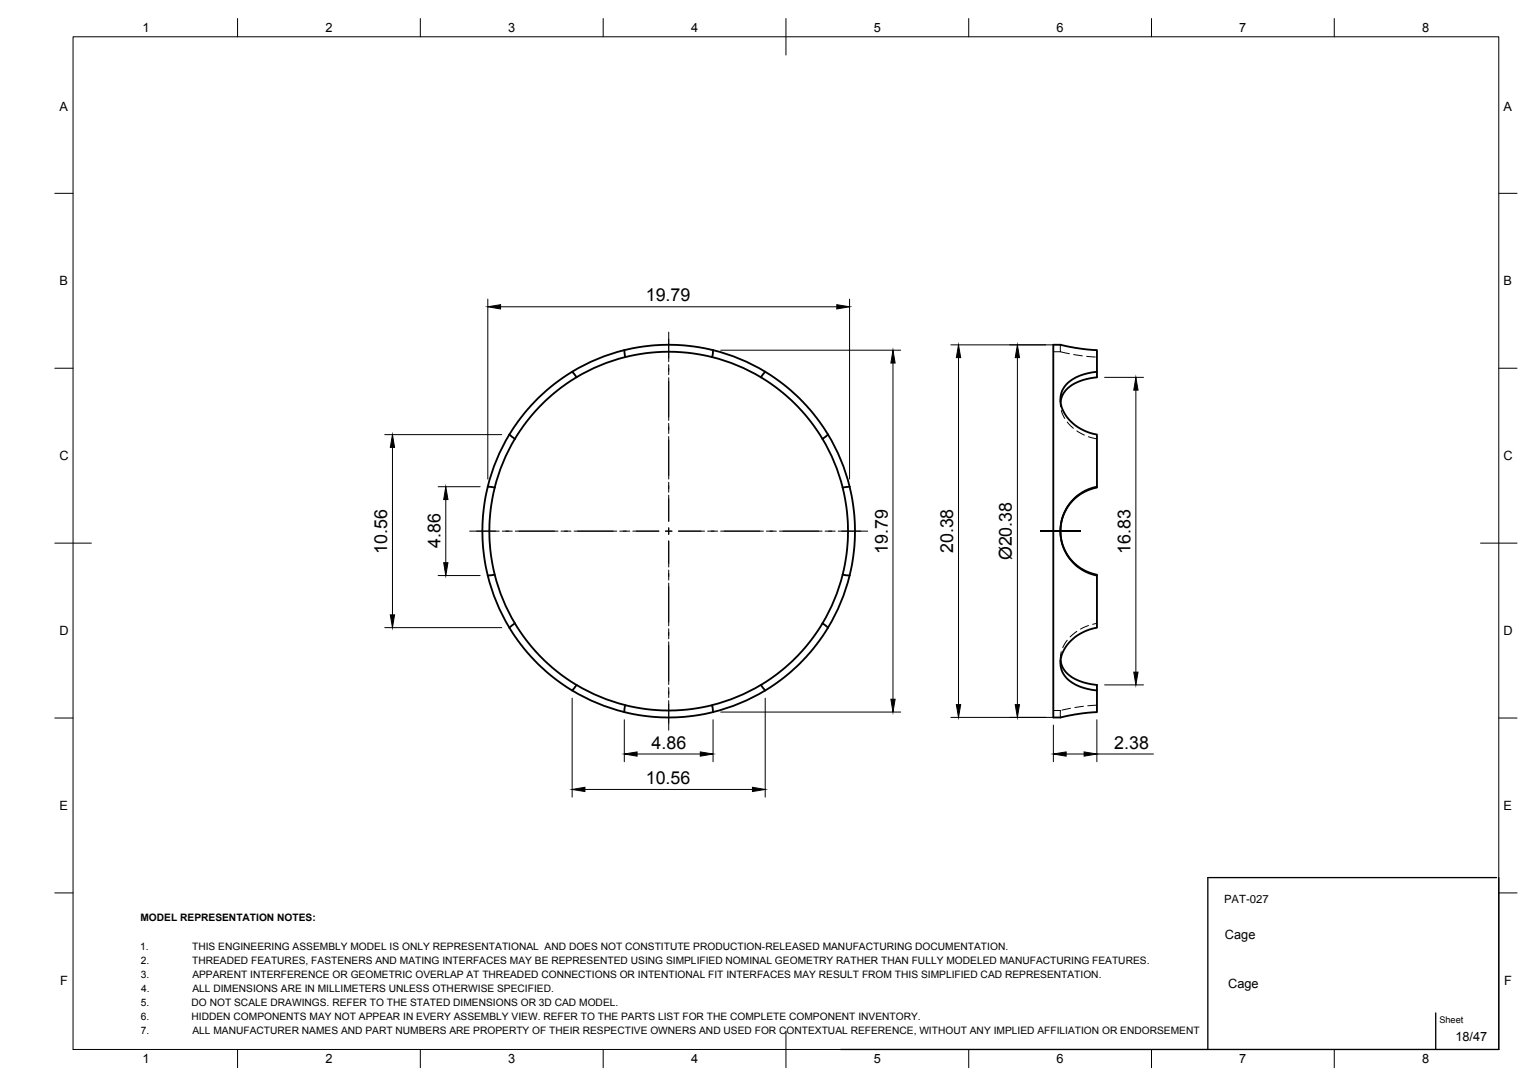
ISO-10303-21;
HEADER;
/* Generated by software containing ST-Developer
 * from STEP Tools, Inc. (www.steptools.com) 
 */

FILE_DESCRIPTION(
/* description */ ('Crank-driven oscillating fan base (mechanism only)'),

/* implementation_level */ '2;1');

FILE_NAME(
/* name */ 'Cage.step',
/* time_stamp */ '2026-10-28T03:25:00-07:00',
/* author */ (''),
/* organization */ (''),
/* preprocessor_version */ 'ST-DEVELOPER v20.2',
/* originating_system */ 'Autodesk Translation Framework v15.17.0.0',
/* authorisation */ '');

FILE_SCHEMA (('AUTOMOTIVE_DESIGN { 1 0 10303 214 3 1 1 }'));
ENDSEC;

DATA;
#10=MECHANICAL_DESIGN_GEOMETRIC_PRESENTATION_REPRESENTATION('',(#456),#11916);
#283=SPHERICAL_SURFACE('',#6888,0.247676);
#284=SPHERICAL_SURFACE('',#6904,0.247676);
#285=SPHERICAL_SURFACE('',#6909,0.247676);
#286=SPHERICAL_SURFACE('',#6914,0.247676);
#287=SPHERICAL_SURFACE('',#6919,0.247676);
#288=SPHERICAL_SURFACE('',#6924,0.247676);
#289=SPHERICAL_SURFACE('',#6929,0.247676);
#290=SPHERICAL_SURFACE('',#6937,0.247676);
#324=B_SPLINE_CURVE_WITH_KNOTS('',3,(#10274,#10275,#10276,#10277,#10278,
#10279,#10280,#10281,#10282,#10283,#10284,#10285,#10286,#10287,#10288,#10289,
#10290,#10291,#10292,#10293,#10294,#10295),.UNSPECIFIED.,.F.,.F.,(4,2,2,
2,2,2,2,2,2,2,4),(0.0473477652366656,0.126350602536658,0.189525903804987,
0.252701205073317,0.313298422430275,0.373895639787233,0.434492857144191,
0.495090074501149,0.558265375769478,0.621440677037807,0.7004435143378),
 .UNSPECIFIED.);
#325=B_SPLINE_CURVE_WITH_KNOTS('',3,(#10299,#10300,#10301,#10302,#10303,
#10304,#10305,#10306,#10307,#10308,#10309,#10310,#10311,#10312,#10313,#10314,
#10315,#10316,#10317,#10318,#10319,#10320),.UNSPECIFIED.,.F.,.F.,(4,2,2,
2,2,2,2,2,2,2,4),(0.0464897534940957,0.0852567806515119,0.170513561303024,
0.246687263103517,0.308657850341199,0.370628437578881,0.432599024816563,
0.494569612054245,0.570743313854739,0.656000094506251,0.694767121663666),
 .UNSPECIFIED.);
#326=B_SPLINE_CURVE_WITH_KNOTS('',3,(#10326,#10327,#10328,#10329,#10330,
#10331,#10332,#10333,#10334,#10335,#10336,#10337,#10338,#10339,#10340,#10341,
#10342,#10343,#10344,#10345,#10346,#10347),.UNSPECIFIED.,.F.,.F.,(4,2,2,
2,2,2,2,2,2,2,4),(0.0464897534940957,0.0852567806515118,0.170513561303024,
0.246687263103517,0.308657850341199,0.370628437578881,0.432599024816563,
0.494569612054245,0.570743313854738,0.65600009450625,0.694767121663666),
 .UNSPECIFIED.);
#327=B_SPLINE_CURVE_WITH_KNOTS('',3,(#10351,#10352,#10353,#10354,#10355,
#10356,#10357,#10358,#10359,#10360,#10361,#10362,#10363,#10364,#10365,#10366,
#10367,#10368,#10369,#10370,#10371,#10372),.UNSPECIFIED.,.F.,.F.,(4,2,2,
2,2,2,2,2,2,2,4),(0.0464897534940957,0.0852567806515119,0.170513561303024,
0.246687263103517,0.308657850341199,0.370628437578881,0.432599024816563,
0.494569612054245,0.570743313854739,0.656000094506251,0.694767121663666),
 .UNSPECIFIED.);
#328=B_SPLINE_CURVE_WITH_KNOTS('',3,(#10376,#10377,#10378,#10379,#10380,
#10381,#10382,#10383,#10384,#10385,#10386,#10387),.UNSPECIFIED.,.F.,.F.,
(4,2,2,2,2,4),(0.0464897534940957,0.0852567806515119,0.170513561303024,
0.246687263103517,0.308657850341199,0.370628437578881),.UNSPECIFIED.);
#329=B_SPLINE_CURVE_WITH_KNOTS('',3,(#10392,#10393,#10394,#10395,#10396,
#10397,#10398,#10399,#10400,#10401,#10402,#10403),.UNSPECIFIED.,.F.,.F.,
(4,2,2,2,2,4),(0.370628437578881,0.432599024816563,0.494569612054245,0.570743313854738,
0.65600009450625,0.694767121663666),.UNSPECIFIED.);
#330=B_SPLINE_CURVE_WITH_KNOTS('',3,(#10407,#10408,#10409,#10410,#10411,
#10412,#10413,#10414,#10415,#10416,#10417,#10418,#10419,#10420,#10421,#10422,
#10423,#10424,#10425,#10426,#10427,#10428),.UNSPECIFIED.,.F.,.F.,(4,2,2,
2,2,2,2,2,2,2,4),(0.0464897534940957,0.0852567806515121,0.170513561303024,
0.246687263103518,0.308657850341199,0.370628437578881,0.432599024816563,
0.494569612054245,0.570743313854738,0.65600009450625,0.694767121663666),
 .UNSPECIFIED.);
#331=B_SPLINE_CURVE_WITH_KNOTS('',3,(#10432,#10433,#10434,#10435,#10436,
#10437,#10438,#10439,#10440,#10441,#10442,#10443,#10444,#10445,#10446,#10447,
#10448,#10449,#10450,#10451,#10452,#10453),.UNSPECIFIED.,.F.,.F.,(4,2,2,
2,2,2,2,2,2,2,4),(0.0464897534940957,0.0852567806515119,0.170513561303024,
0.246687263103517,0.308657850341199,0.370628437578881,0.432599024816563,
0.494569612054245,0.570743313854738,0.65600009450625,0.694767121663667),
 .UNSPECIFIED.);
#332=B_SPLINE_CURVE_WITH_KNOTS('',3,(#10457,#10458,#10459,#10460,#10461,
#10462,#10463,#10464,#10465,#10466,#10467,#10468,#10469,#10470,#10471,#10472,
#10473,#10474,#10475,#10476,#10477,#10478),.UNSPECIFIED.,.F.,.F.,(4,2,2,
2,2,2,2,2,2,2,4),(0.0464897534940957,0.0852567806515119,0.170513561303024,
0.246687263103517,0.308657850341199,0.370628437578881,0.432599024816563,
0.494569612054245,0.570743313854738,0.65600009450625,0.694767121663666),
 .UNSPECIFIED.);
#333=B_SPLINE_CURVE_WITH_KNOTS('',3,(#10482,#10483,#10484,#10485,#10486,
#10487,#10488,#10489,#10490,#10491,#10492,#10493,#10494,#10495,#10496,#10497,
#10498,#10499,#10500,#10501,#10502,#10503),.UNSPECIFIED.,.F.,.F.,(4,2,2,
2,2,2,2,2,2,2,4),(0.0464897534940957,0.0852567806515119,0.170513561303024,
0.246687263103517,0.308657850341199,0.370628437578881,0.432599024816563,
0.494569612054245,0.570743313854739,0.656000094506251,0.694767121663667),
 .UNSPECIFIED.);
#334=B_SPLINE_CURVE_WITH_KNOTS('',3,(#10511,#10512,#10513,#10514,#10515,
#10516,#10517,#10518,#10519,#10520,#10521,#10522,#10523,#10524,#10525,#10526,
#10527,#10528,#10529,#10530,#10531,#10532),.UNSPECIFIED.,.F.,.F.,(4,2,2,
2,2,2,2,2,2,2,4),(0.0473477652366656,0.126350602536658,0.189525903804987,
0.252701205073316,0.313298422430274,0.373895639787232,0.434492857144191,
0.495090074501149,0.558265375769478,0.621440677037807,0.7004435143378),
 .UNSPECIFIED.);
#335=B_SPLINE_CURVE_WITH_KNOTS('',3,(#10540,#10541,#10542,#10543,#10544,
#10545,#10546,#10547,#10548,#10549,#10550,#10551,#10552,#10553,#10554,#10555,
#10556,#10557,#10558,#10559,#10560,#10561),.UNSPECIFIED.,.F.,.F.,(4,2,2,
2,2,2,2,2,2,2,4),(0.0473477652366656,0.126350602536658,0.189525903804987,
0.252701205073317,0.313298422430275,0.373895639787233,0.434492857144191,
0.495090074501149,0.558265375769478,0.621440677037807,0.7004435143378),
 .UNSPECIFIED.);
#336=B_SPLINE_CURVE_WITH_KNOTS('',3,(#10570,#10571,#10572,#10573,#10574,
#10575,#10576,#10577,#10578,#10579,#10580,#10581),.UNSPECIFIED.,.F.,.F.,
(4,2,2,2,2,4),(0.0473477652366656,0.126350602536658,0.189525903804987,0.252701205073316,
0.313298422430275,0.373895639787233),.UNSPECIFIED.);
#337=B_SPLINE_CURVE_WITH_KNOTS('',3,(#10583,#10584,#10585,#10586,#10587,
#10588,#10589,#10590,#10591,#10592,#10593,#10594),.UNSPECIFIED.,.F.,.F.,
(4,2,2,2,2,4),(0.373895639787233,0.434492857144191,0.495090074501149,0.558265375769478,
0.621440677037807,0.7004435143378),.UNSPECIFIED.);
#338=B_SPLINE_CURVE_WITH_KNOTS('',3,(#10601,#10602,#10603,#10604,#10605,
#10606,#10607,#10608,#10609,#10610,#10611,#10612,#10613,#10614,#10615,#10616,
#10617,#10618,#10619,#10620,#10621,#10622),.UNSPECIFIED.,.F.,.F.,(4,2,2,
2,2,2,2,2,2,2,4),(0.0473477652366656,0.126350602536658,0.189525903804987,
0.252701205073316,0.313298422430275,0.373895639787233,0.434492857144191,
0.495090074501149,0.558265375769478,0.621440677037807,0.7004435143378),
 .UNSPECIFIED.);
#339=B_SPLINE_CURVE_WITH_KNOTS('',3,(#10630,#10631,#10632,#10633,#10634,
#10635,#10636,#10637,#10638,#10639,#10640,#10641,#10642,#10643,#10644,#10645,
#10646,#10647,#10648,#10649,#10650,#10651),.UNSPECIFIED.,.F.,.F.,(4,2,2,
2,2,2,2,2,2,2,4),(0.0473477652366656,0.126350602536658,0.189525903804987,
0.252701205073317,0.313298422430275,0.373895639787233,0.434492857144191,
0.495090074501149,0.558265375769478,0.621440677037807,0.7004435143378),
 .UNSPECIFIED.);
#340=B_SPLINE_CURVE_WITH_KNOTS('',3,(#10659,#10660,#10661,#10662,#10663,
#10664,#10665,#10666,#10667,#10668,#10669,#10670,#10671,#10672,#10673,#10674,
#10675,#10676,#10677,#10678,#10679,#10680),.UNSPECIFIED.,.F.,.F.,(4,2,2,
2,2,2,2,2,2,2,4),(0.0473477652366656,0.126350602536658,0.189525903804987,
0.252701205073316,0.313298422430275,0.373895639787233,0.434492857144191,
0.495090074501149,0.558265375769478,0.621440677037807,0.7004435143378),
 .UNSPECIFIED.);
#341=B_SPLINE_CURVE_WITH_KNOTS('',3,(#10689,#10690,#10691,#10692,#10693,
#10694,#10695,#10696,#10697,#10698,#10699,#10700,#10701,#10702,#10703,#10704,
#10705,#10706,#10707,#10708,#10709,#10710),.UNSPECIFIED.,.F.,.F.,(4,2,2,
2,2,2,2,2,2,2,4),(0.0473477652366656,0.126350602536658,0.189525903804987,
0.252701205073317,0.313298422430275,0.373895639787233,0.434492857144191,
0.495090074501149,0.558265375769478,0.621440677037807,0.7004435143378),
 .UNSPECIFIED.);
#369=SHAPE_REPRESENTATION_RELATIONSHIP('SRR','None',#12094,#409);
#409=ADVANCED_BREP_SHAPE_REPRESENTATION('',(#503),#11885);
#456=STYLED_ITEM('',(#12375),#503);
#503=MANIFOLD_SOLID_BREP('Continuous crown cage',#6087);
#611=FACE_BOUND('',#1508,.T.);
#757=PLANE('',#6901);
#758=PLANE('',#6906);
#759=PLANE('',#6911);
#760=PLANE('',#6916);
#761=PLANE('',#6921);
#762=PLANE('',#6926);
#763=PLANE('',#6935);
#764=PLANE('',#6939);
#765=PLANE('',#6940);
#1034=FACE_OUTER_BOUND('',#1490,.T.);
#1035=FACE_OUTER_BOUND('',#1491,.T.);
#1036=FACE_OUTER_BOUND('',#1492,.T.);
#1037=FACE_OUTER_BOUND('',#1493,.T.);
#1038=FACE_OUTER_BOUND('',#1494,.T.);
#1039=FACE_OUTER_BOUND('',#1495,.T.);
#1040=FACE_OUTER_BOUND('',#1496,.T.);
#1041=FACE_OUTER_BOUND('',#1497,.T.);
#1042=FACE_OUTER_BOUND('',#1498,.T.);
#1043=FACE_OUTER_BOUND('',#1499,.T.);
#1044=FACE_OUTER_BOUND('',#1500,.T.);
#1045=FACE_OUTER_BOUND('',#1501,.T.);
#1046=FACE_OUTER_BOUND('',#1502,.T.);
#1047=FACE_OUTER_BOUND('',#1503,.T.);
#1048=FACE_OUTER_BOUND('',#1504,.T.);
#1049=FACE_OUTER_BOUND('',#1505,.T.);
#1050=FACE_OUTER_BOUND('',#1506,.T.);
#1051=FACE_OUTER_BOUND('',#1507,.T.);
#1052=FACE_OUTER_BOUND('',#1509,.T.);
#1490=EDGE_LOOP('',(#4684,#4685,#4686,#4687));
#1491=EDGE_LOOP('',(#4688,#4689,#4690,#4691,#4692,#4693,#4694,#4695,#4696,
#4697,#4698,#4699,#4700,#4701,#4702,#4703,#4704,#4705,#4706,#4707));
#1492=EDGE_LOOP('',(#4708,#4709,#4710,#4711));
#1493=EDGE_LOOP('',(#4712,#4713,#4714,#4715));
#1494=EDGE_LOOP('',(#4716,#4717,#4718,#4719));
#1495=EDGE_LOOP('',(#4720,#4721,#4722,#4723));
#1496=EDGE_LOOP('',(#4724,#4725,#4726,#4727));
#1497=EDGE_LOOP('',(#4728,#4729,#4730,#4731,#4732,#4733));
#1498=EDGE_LOOP('',(#4734,#4735,#4736,#4737));
#1499=EDGE_LOOP('',(#4738,#4739,#4740,#4741));
#1500=EDGE_LOOP('',(#4742,#4743,#4744,#4745));
#1501=EDGE_LOOP('',(#4746,#4747,#4748,#4749));
#1502=EDGE_LOOP('',(#4750,#4751,#4752,#4753));
#1503=EDGE_LOOP('',(#4754,#4755,#4756,#4757));
#1504=EDGE_LOOP('',(#4758,#4759,#4760,#4761,#4762,#4763,#4764,#4765,#4766,
#4767,#4768,#4769,#4770,#4771,#4772,#4773,#4774,#4775,#4776,#4777));
#1505=EDGE_LOOP('',(#4778,#4779,#4780,#4781));
#1506=EDGE_LOOP('',(#4782,#4783,#4784,#4785));
#1507=EDGE_LOOP('',(#4786));
#1508=EDGE_LOOP('',(#4787));
#1509=EDGE_LOOP('',(#4788,#4789,#4790,#4791));
#1933=LINE('',#10389,#2266);
#1934=LINE('',#10685,#2267);
#2266=VECTOR('',#8218,1.019052);
#2267=VECTOR('',#8295,0.980948);
#2629=CIRCLE('',#6889,0.243053047864041);
#2630=CIRCLE('',#6890,0.243053047864041);
#2631=CIRCLE('',#6892,1.019052);
#2632=CIRCLE('',#6893,1.019052);
#2633=CIRCLE('',#6894,1.019052);
#2634=CIRCLE('',#6895,1.019052);
#2635=CIRCLE('',#6896,1.019052);
#2636=CIRCLE('',#6897,1.019052);
#2637=CIRCLE('',#6898,1.019052);
#2638=CIRCLE('',#6899,1.019052);
#2639=CIRCLE('',#6900,1.019052);
#2640=CIRCLE('',#6902,0.980948);
#2641=CIRCLE('',#6903,0.243053047864041);
#2642=CIRCLE('',#6905,0.243053047864041);
#2643=CIRCLE('',#6907,0.980948);
#2644=CIRCLE('',#6908,0.243053047864041);
#2645=CIRCLE('',#6910,0.243053047864041);
#2646=CIRCLE('',#6912,0.980948);
#2647=CIRCLE('',#6913,0.243053047864041);
#2648=CIRCLE('',#6915,0.243053047864041);
#2649=CIRCLE('',#6917,0.980948);
#2650=CIRCLE('',#6918,0.243053047864041);
#2651=CIRCLE('',#6920,0.243053047864041);
#2652=CIRCLE('',#6922,0.980948);
#2653=CIRCLE('',#6923,0.243053047864041);
#2654=CIRCLE('',#6925,0.243053047864041);
#2655=CIRCLE('',#6927,0.980948);
#2656=CIRCLE('',#6928,0.243053047864041);
#2657=CIRCLE('',#6930,0.243053047864041);
#2658=CIRCLE('',#6932,0.980948);
#2659=CIRCLE('',#6933,0.980948);
#2660=CIRCLE('',#6934,0.980948);
#2661=CIRCLE('',#6936,0.243053047864041);
#2662=CIRCLE('',#6938,0.243053047864041);
#3044=VERTEX_POINT('',#10272);
#3045=VERTEX_POINT('',#10273);
#3046=VERTEX_POINT('',#10296);
#3047=VERTEX_POINT('',#10298);
#3048=VERTEX_POINT('',#10323);
#3049=VERTEX_POINT('',#10325);
#3050=VERTEX_POINT('',#10348);
#3051=VERTEX_POINT('',#10350);
#3052=VERTEX_POINT('',#10373);
#3053=VERTEX_POINT('',#10375);
#3054=VERTEX_POINT('',#10388);
#3055=VERTEX_POINT('',#10391);
#3056=VERTEX_POINT('',#10404);
#3057=VERTEX_POINT('',#10406);
#3058=VERTEX_POINT('',#10429);
#3059=VERTEX_POINT('',#10431);
#3060=VERTEX_POINT('',#10454);
#3061=VERTEX_POINT('',#10456);
#3062=VERTEX_POINT('',#10479);
#3063=VERTEX_POINT('',#10481);
#3064=VERTEX_POINT('',#10506);
#3065=VERTEX_POINT('',#10510);
#3066=VERTEX_POINT('',#10535);
#3067=VERTEX_POINT('',#10539);
#3068=VERTEX_POINT('',#10564);
#3069=VERTEX_POINT('',#10568);
#3070=VERTEX_POINT('',#10569);
#3071=VERTEX_POINT('',#10596);
#3072=VERTEX_POINT('',#10600);
#3073=VERTEX_POINT('',#10625);
#3074=VERTEX_POINT('',#10629);
#3075=VERTEX_POINT('',#10654);
#3076=VERTEX_POINT('',#10658);
#3077=VERTEX_POINT('',#10683);
#3078=VERTEX_POINT('',#10686);
#3079=VERTEX_POINT('',#10688);
#3637=EDGE_CURVE('',#3044,#3045,#324,.T.);
#3638=EDGE_CURVE('',#3046,#3044,#2629,.T.);
#3639=EDGE_CURVE('',#3047,#3046,#325,.T.);
#3640=EDGE_CURVE('',#3045,#3047,#2630,.T.);
#3641=EDGE_CURVE('',#3048,#3046,#2631,.T.);
#3642=EDGE_CURVE('',#3048,#3049,#326,.T.);
#3643=EDGE_CURVE('',#3050,#3049,#2632,.T.);
#3644=EDGE_CURVE('',#3050,#3051,#327,.T.);
#3645=EDGE_CURVE('',#3052,#3051,#2633,.T.);
#3646=EDGE_CURVE('',#3052,#3053,#328,.T.);
#3647=EDGE_CURVE('',#3053,#3054,#1933,.T.);
#3648=EDGE_CURVE('',#3054,#3054,#2634,.T.);
#3649=EDGE_CURVE('',#3053,#3055,#329,.T.);
#3650=EDGE_CURVE('',#3056,#3055,#2635,.T.);
#3651=EDGE_CURVE('',#3056,#3057,#330,.T.);
#3652=EDGE_CURVE('',#3058,#3057,#2636,.T.);
#3653=EDGE_CURVE('',#3058,#3059,#331,.T.);
#3654=EDGE_CURVE('',#3060,#3059,#2637,.T.);
#3655=EDGE_CURVE('',#3060,#3061,#332,.T.);
#3656=EDGE_CURVE('',#3062,#3061,#2638,.T.);
#3657=EDGE_CURVE('',#3062,#3063,#333,.T.);
#3658=EDGE_CURVE('',#3047,#3063,#2639,.T.);
#3659=EDGE_CURVE('',#3044,#3064,#2640,.T.);
#3660=EDGE_CURVE('',#3064,#3048,#2641,.T.);
#3661=EDGE_CURVE('',#3065,#3064,#334,.T.);
#3662=EDGE_CURVE('',#3049,#3065,#2642,.T.);
#3663=EDGE_CURVE('',#3065,#3066,#2643,.T.);
#3664=EDGE_CURVE('',#3066,#3050,#2644,.T.);
#3665=EDGE_CURVE('',#3067,#3066,#335,.T.);
#3666=EDGE_CURVE('',#3051,#3067,#2645,.T.);
#3667=EDGE_CURVE('',#3067,#3068,#2646,.T.);
#3668=EDGE_CURVE('',#3068,#3052,#2647,.T.);
#3669=EDGE_CURVE('',#3069,#3070,#336,.T.);
#3670=EDGE_CURVE('',#3055,#3069,#2648,.T.);
#3671=EDGE_CURVE('',#3070,#3068,#337,.T.);
#3672=EDGE_CURVE('',#3069,#3071,#2649,.T.);
#3673=EDGE_CURVE('',#3071,#3056,#2650,.T.);
#3674=EDGE_CURVE('',#3072,#3071,#338,.T.);
#3675=EDGE_CURVE('',#3057,#3072,#2651,.T.);
#3676=EDGE_CURVE('',#3072,#3073,#2652,.T.);
#3677=EDGE_CURVE('',#3073,#3058,#2653,.T.);
#3678=EDGE_CURVE('',#3074,#3073,#339,.T.);
#3679=EDGE_CURVE('',#3059,#3074,#2654,.T.);
#3680=EDGE_CURVE('',#3074,#3075,#2655,.T.);
#3681=EDGE_CURVE('',#3075,#3060,#2656,.T.);
#3682=EDGE_CURVE('',#3076,#3075,#340,.T.);
#3683=EDGE_CURVE('',#3061,#3076,#2657,.T.);
#3684=EDGE_CURVE('',#3077,#3077,#2658,.T.);
#3685=EDGE_CURVE('',#3077,#3070,#1934,.T.);
#3686=EDGE_CURVE('',#3078,#3045,#2659,.T.);
#3687=EDGE_CURVE('',#3078,#3079,#341,.T.);
#3688=EDGE_CURVE('',#3076,#3079,#2660,.T.);
#3689=EDGE_CURVE('',#3063,#3078,#2661,.T.);
#3690=EDGE_CURVE('',#3079,#3062,#2662,.T.);
#4684=ORIENTED_EDGE('',*,*,#3637,.F.);
#4685=ORIENTED_EDGE('',*,*,#3638,.F.);
#4686=ORIENTED_EDGE('',*,*,#3639,.F.);
#4687=ORIENTED_EDGE('',*,*,#3640,.F.);
#4688=ORIENTED_EDGE('',*,*,#3639,.T.);
#4689=ORIENTED_EDGE('',*,*,#3641,.F.);
#4690=ORIENTED_EDGE('',*,*,#3642,.T.);
#4691=ORIENTED_EDGE('',*,*,#3643,.F.);
#4692=ORIENTED_EDGE('',*,*,#3644,.T.);
#4693=ORIENTED_EDGE('',*,*,#3645,.F.);
#4694=ORIENTED_EDGE('',*,*,#3646,.T.);
#4695=ORIENTED_EDGE('',*,*,#3647,.T.);
#4696=ORIENTED_EDGE('',*,*,#3648,.F.);
#4697=ORIENTED_EDGE('',*,*,#3647,.F.);
#4698=ORIENTED_EDGE('',*,*,#3649,.T.);
#4699=ORIENTED_EDGE('',*,*,#3650,.F.);
#4700=ORIENTED_EDGE('',*,*,#3651,.T.);
#4701=ORIENTED_EDGE('',*,*,#3652,.F.);
#4702=ORIENTED_EDGE('',*,*,#3653,.T.);
#4703=ORIENTED_EDGE('',*,*,#3654,.F.);
#4704=ORIENTED_EDGE('',*,*,#3655,.T.);
#4705=ORIENTED_EDGE('',*,*,#3656,.F.);
#4706=ORIENTED_EDGE('',*,*,#3657,.T.);
#4707=ORIENTED_EDGE('',*,*,#3658,.F.);
#4708=ORIENTED_EDGE('',*,*,#3638,.T.);
#4709=ORIENTED_EDGE('',*,*,#3659,.T.);
#4710=ORIENTED_EDGE('',*,*,#3660,.T.);
#4711=ORIENTED_EDGE('',*,*,#3641,.T.);
#4712=ORIENTED_EDGE('',*,*,#3661,.F.);
#4713=ORIENTED_EDGE('',*,*,#3662,.F.);
#4714=ORIENTED_EDGE('',*,*,#3642,.F.);
#4715=ORIENTED_EDGE('',*,*,#3660,.F.);
#4716=ORIENTED_EDGE('',*,*,#3662,.T.);
#4717=ORIENTED_EDGE('',*,*,#3663,.T.);
#4718=ORIENTED_EDGE('',*,*,#3664,.T.);
#4719=ORIENTED_EDGE('',*,*,#3643,.T.);
#4720=ORIENTED_EDGE('',*,*,#3665,.F.);
#4721=ORIENTED_EDGE('',*,*,#3666,.F.);
#4722=ORIENTED_EDGE('',*,*,#3644,.F.);
#4723=ORIENTED_EDGE('',*,*,#3664,.F.);
#4724=ORIENTED_EDGE('',*,*,#3666,.T.);
#4725=ORIENTED_EDGE('',*,*,#3667,.T.);
#4726=ORIENTED_EDGE('',*,*,#3668,.T.);
#4727=ORIENTED_EDGE('',*,*,#3645,.T.);
#4728=ORIENTED_EDGE('',*,*,#3669,.F.);
#4729=ORIENTED_EDGE('',*,*,#3670,.F.);
#4730=ORIENTED_EDGE('',*,*,#3649,.F.);
#4731=ORIENTED_EDGE('',*,*,#3646,.F.);
#4732=ORIENTED_EDGE('',*,*,#3668,.F.);
#4733=ORIENTED_EDGE('',*,*,#3671,.F.);
#4734=ORIENTED_EDGE('',*,*,#3670,.T.);
#4735=ORIENTED_EDGE('',*,*,#3672,.T.);
#4736=ORIENTED_EDGE('',*,*,#3673,.T.);
#4737=ORIENTED_EDGE('',*,*,#3650,.T.);
#4738=ORIENTED_EDGE('',*,*,#3674,.F.);
#4739=ORIENTED_EDGE('',*,*,#3675,.F.);
#4740=ORIENTED_EDGE('',*,*,#3651,.F.);
#4741=ORIENTED_EDGE('',*,*,#3673,.F.);
#4742=ORIENTED_EDGE('',*,*,#3675,.T.);
#4743=ORIENTED_EDGE('',*,*,#3676,.T.);
#4744=ORIENTED_EDGE('',*,*,#3677,.T.);
#4745=ORIENTED_EDGE('',*,*,#3652,.T.);
#4746=ORIENTED_EDGE('',*,*,#3678,.F.);
#4747=ORIENTED_EDGE('',*,*,#3679,.F.);
#4748=ORIENTED_EDGE('',*,*,#3653,.F.);
#4749=ORIENTED_EDGE('',*,*,#3677,.F.);
#4750=ORIENTED_EDGE('',*,*,#3679,.T.);
#4751=ORIENTED_EDGE('',*,*,#3680,.T.);
#4752=ORIENTED_EDGE('',*,*,#3681,.T.);
#4753=ORIENTED_EDGE('',*,*,#3654,.T.);
#4754=ORIENTED_EDGE('',*,*,#3655,.F.);
#4755=ORIENTED_EDGE('',*,*,#3681,.F.);
#4756=ORIENTED_EDGE('',*,*,#3682,.F.);
#4757=ORIENTED_EDGE('',*,*,#3683,.F.);
#4758=ORIENTED_EDGE('',*,*,#3684,.F.);
#4759=ORIENTED_EDGE('',*,*,#3685,.T.);
#4760=ORIENTED_EDGE('',*,*,#3671,.T.);
#4761=ORIENTED_EDGE('',*,*,#3667,.F.);
#4762=ORIENTED_EDGE('',*,*,#3665,.T.);
#4763=ORIENTED_EDGE('',*,*,#3663,.F.);
#4764=ORIENTED_EDGE('',*,*,#3661,.T.);
#4765=ORIENTED_EDGE('',*,*,#3659,.F.);
#4766=ORIENTED_EDGE('',*,*,#3637,.T.);
#4767=ORIENTED_EDGE('',*,*,#3686,.F.);
#4768=ORIENTED_EDGE('',*,*,#3687,.T.);
#4769=ORIENTED_EDGE('',*,*,#3688,.F.);
#4770=ORIENTED_EDGE('',*,*,#3682,.T.);
#4771=ORIENTED_EDGE('',*,*,#3680,.F.);
#4772=ORIENTED_EDGE('',*,*,#3678,.T.);
#4773=ORIENTED_EDGE('',*,*,#3676,.F.);
#4774=ORIENTED_EDGE('',*,*,#3674,.T.);
#4775=ORIENTED_EDGE('',*,*,#3672,.F.);
#4776=ORIENTED_EDGE('',*,*,#3669,.T.);
#4777=ORIENTED_EDGE('',*,*,#3685,.F.);
#4778=ORIENTED_EDGE('',*,*,#3640,.T.);
#4779=ORIENTED_EDGE('',*,*,#3658,.T.);
#4780=ORIENTED_EDGE('',*,*,#3689,.T.);
#4781=ORIENTED_EDGE('',*,*,#3686,.T.);
#4782=ORIENTED_EDGE('',*,*,#3657,.F.);
#4783=ORIENTED_EDGE('',*,*,#3690,.F.);
#4784=ORIENTED_EDGE('',*,*,#3687,.F.);
#4785=ORIENTED_EDGE('',*,*,#3689,.F.);
#4786=ORIENTED_EDGE('',*,*,#3648,.T.);
#4787=ORIENTED_EDGE('',*,*,#3684,.T.);
#4788=ORIENTED_EDGE('',*,*,#3683,.T.);
#4789=ORIENTED_EDGE('',*,*,#3688,.T.);
#4790=ORIENTED_EDGE('',*,*,#3690,.T.);
#4791=ORIENTED_EDGE('',*,*,#3656,.T.);
#5612=CYLINDRICAL_SURFACE('',#6891,1.019052);
#5613=CYLINDRICAL_SURFACE('',#6931,0.980948);
#5840=ADVANCED_FACE('',(#1034),#283,.F.);
#5841=ADVANCED_FACE('',(#1035),#5612,.T.);
#5842=ADVANCED_FACE('',(#1036),#757,.T.);
#5843=ADVANCED_FACE('',(#1037),#284,.F.);
#5844=ADVANCED_FACE('',(#1038),#758,.T.);
#5845=ADVANCED_FACE('',(#1039),#285,.F.);
#5846=ADVANCED_FACE('',(#1040),#759,.T.);
#5847=ADVANCED_FACE('',(#1041),#286,.F.);
#5848=ADVANCED_FACE('',(#1042),#760,.T.);
#5849=ADVANCED_FACE('',(#1043),#287,.F.);
#5850=ADVANCED_FACE('',(#1044),#761,.T.);
#5851=ADVANCED_FACE('',(#1045),#288,.F.);
#5852=ADVANCED_FACE('',(#1046),#762,.T.);
#5853=ADVANCED_FACE('',(#1047),#289,.F.);
#5854=ADVANCED_FACE('',(#1048),#5613,.F.);
#5855=ADVANCED_FACE('',(#1049),#763,.T.);
#5856=ADVANCED_FACE('',(#1050),#290,.F.);
#5857=ADVANCED_FACE('',(#1051,#611),#764,.T.);
#5858=ADVANCED_FACE('',(#1052),#765,.T.);
#6087=CLOSED_SHELL('',(#5840,#5841,#5842,#5843,#5844,#5845,#5846,#5847,
#5848,#5849,#5850,#5851,#5852,#5853,#5854,#5855,#5856,#5857,#5858));
#6887=AXIS2_PLACEMENT_3D('',#10270,#8202,#8203);
#6888=AXIS2_PLACEMENT_3D('',#10271,#8204,#8205);
#6889=AXIS2_PLACEMENT_3D('',#10297,#8206,#8207);
#6890=AXIS2_PLACEMENT_3D('',#10321,#8208,#8209);
#6891=AXIS2_PLACEMENT_3D('',#10322,#8210,#8211);
#6892=AXIS2_PLACEMENT_3D('',#10324,#8212,#8213);
#6893=AXIS2_PLACEMENT_3D('',#10349,#8214,#8215);
#6894=AXIS2_PLACEMENT_3D('',#10374,#8216,#8217);
#6895=AXIS2_PLACEMENT_3D('',#10390,#8219,#8220);
#6896=AXIS2_PLACEMENT_3D('',#10405,#8221,#8222);
#6897=AXIS2_PLACEMENT_3D('',#10430,#8223,#8224);
#6898=AXIS2_PLACEMENT_3D('',#10455,#8225,#8226);
#6899=AXIS2_PLACEMENT_3D('',#10480,#8227,#8228);
#6900=AXIS2_PLACEMENT_3D('',#10504,#8229,#8230);
#6901=AXIS2_PLACEMENT_3D('',#10505,#8231,#8232);
#6902=AXIS2_PLACEMENT_3D('',#10507,#8233,#8234);
#6903=AXIS2_PLACEMENT_3D('',#10508,#8235,#8236);
#6904=AXIS2_PLACEMENT_3D('',#10509,#8237,#8238);
#6905=AXIS2_PLACEMENT_3D('',#10533,#8239,#8240);
#6906=AXIS2_PLACEMENT_3D('',#10534,#8241,#8242);
#6907=AXIS2_PLACEMENT_3D('',#10536,#8243,#8244);
#6908=AXIS2_PLACEMENT_3D('',#10537,#8245,#8246);
#6909=AXIS2_PLACEMENT_3D('',#10538,#8247,#8248);
#6910=AXIS2_PLACEMENT_3D('',#10562,#8249,#8250);
#6911=AXIS2_PLACEMENT_3D('',#10563,#8251,#8252);
#6912=AXIS2_PLACEMENT_3D('',#10565,#8253,#8254);
#6913=AXIS2_PLACEMENT_3D('',#10566,#8255,#8256);
#6914=AXIS2_PLACEMENT_3D('',#10567,#8257,#8258);
#6915=AXIS2_PLACEMENT_3D('',#10582,#8259,#8260);
#6916=AXIS2_PLACEMENT_3D('',#10595,#8261,#8262);
#6917=AXIS2_PLACEMENT_3D('',#10597,#8263,#8264);
#6918=AXIS2_PLACEMENT_3D('',#10598,#8265,#8266);
#6919=AXIS2_PLACEMENT_3D('',#10599,#8267,#8268);
#6920=AXIS2_PLACEMENT_3D('',#10623,#8269,#8270);
#6921=AXIS2_PLACEMENT_3D('',#10624,#8271,#8272);
#6922=AXIS2_PLACEMENT_3D('',#10626,#8273,#8274);
#6923=AXIS2_PLACEMENT_3D('',#10627,#8275,#8276);
#6924=AXIS2_PLACEMENT_3D('',#10628,#8277,#8278);
#6925=AXIS2_PLACEMENT_3D('',#10652,#8279,#8280);
#6926=AXIS2_PLACEMENT_3D('',#10653,#8281,#8282);
#6927=AXIS2_PLACEMENT_3D('',#10655,#8283,#8284);
#6928=AXIS2_PLACEMENT_3D('',#10656,#8285,#8286);
#6929=AXIS2_PLACEMENT_3D('',#10657,#8287,#8288);
#6930=AXIS2_PLACEMENT_3D('',#10681,#8289,#8290);
#6931=AXIS2_PLACEMENT_3D('',#10682,#8291,#8292);
#6932=AXIS2_PLACEMENT_3D('',#10684,#8293,#8294);
#6933=AXIS2_PLACEMENT_3D('',#10687,#8296,#8297);
#6934=AXIS2_PLACEMENT_3D('',#10711,#8298,#8299);
#6935=AXIS2_PLACEMENT_3D('',#10712,#8300,#8301);
#6936=AXIS2_PLACEMENT_3D('',#10713,#8302,#8303);
#6937=AXIS2_PLACEMENT_3D('',#10714,#8304,#8305);
#6938=AXIS2_PLACEMENT_3D('',#10715,#8306,#8307);
#6939=AXIS2_PLACEMENT_3D('',#10716,#8308,#8309);
#6940=AXIS2_PLACEMENT_3D('',#10717,#8310,#8311);
#8202=DIRECTION('axis',(0.,0.,1.));
#8203=DIRECTION('refdir',(1.,0.,0.));
#8204=DIRECTION('center_axis',(0.,0.,1.));
#8205=DIRECTION('ref_axis',(1.,0.,0.));
#8206=DIRECTION('center_axis',(0.,-1.,0.));
#8207=DIRECTION('ref_axis',(0.,0.,-1.));
#8208=DIRECTION('center_axis',(0.,-1.,0.));
#8209=DIRECTION('ref_axis',(0.,0.,-1.));
#8210=DIRECTION('center_axis',(0.,1.,0.));
#8211=DIRECTION('ref_axis',(1.,0.,0.));
#8212=DIRECTION('center_axis',(0.,1.,0.));
#8213=DIRECTION('ref_axis',(1.,0.,0.));
#8214=DIRECTION('center_axis',(0.,1.,0.));
#8215=DIRECTION('ref_axis',(1.,0.,0.));
#8216=DIRECTION('center_axis',(0.,1.,0.));
#8217=DIRECTION('ref_axis',(1.,0.,0.));
#8218=DIRECTION('',(0.,-1.,0.));
#8219=DIRECTION('center_axis',(0.,-1.,0.));
#8220=DIRECTION('ref_axis',(1.,0.,0.));
#8221=DIRECTION('center_axis',(0.,1.,0.));
#8222=DIRECTION('ref_axis',(1.,0.,0.));
#8223=DIRECTION('center_axis',(0.,1.,0.));
#8224=DIRECTION('ref_axis',(1.,0.,0.));
#8225=DIRECTION('center_axis',(0.,1.,0.));
#8226=DIRECTION('ref_axis',(1.,0.,0.));
#8227=DIRECTION('center_axis',(0.,1.,0.));
#8228=DIRECTION('ref_axis',(1.,0.,0.));
#8229=DIRECTION('center_axis',(0.,1.,0.));
#8230=DIRECTION('ref_axis',(1.,0.,0.));
#8231=DIRECTION('center_axis',(0.,1.,0.));
#8232=DIRECTION('ref_axis',(1.,0.,0.));
#8233=DIRECTION('center_axis',(0.,-1.,0.));
#8234=DIRECTION('ref_axis',(1.,0.,0.));
#8235=DIRECTION('center_axis',(0.,-1.,0.));
#8236=DIRECTION('ref_axis',(0.,0.,-1.));
#8237=DIRECTION('center_axis',(6.12323399573677E-17,0.,1.));
#8238=DIRECTION('ref_axis',(1.,0.,0.));
#8239=DIRECTION('center_axis',(0.,-1.,0.));
#8240=DIRECTION('ref_axis',(0.,0.,-1.));
#8241=DIRECTION('center_axis',(0.,1.,0.));
#8242=DIRECTION('ref_axis',(1.,0.,0.));
#8243=DIRECTION('center_axis',(0.,-1.,0.));
#8244=DIRECTION('ref_axis',(1.,0.,0.));
#8245=DIRECTION('center_axis',(0.,-1.,0.));
#8246=DIRECTION('ref_axis',(0.,0.,-1.));
#8247=DIRECTION('center_axis',(0.,0.,1.));
#8248=DIRECTION('ref_axis',(1.,0.,0.));
#8249=DIRECTION('center_axis',(0.,-1.,0.));
#8250=DIRECTION('ref_axis',(0.,0.,-1.));
#8251=DIRECTION('center_axis',(0.,1.,0.));
#8252=DIRECTION('ref_axis',(1.,0.,0.));
#8253=DIRECTION('center_axis',(0.,-1.,0.));
#8254=DIRECTION('ref_axis',(1.,0.,0.));
#8255=DIRECTION('center_axis',(0.,-1.,0.));
#8256=DIRECTION('ref_axis',(0.,0.,-1.));
#8257=DIRECTION('center_axis',(0.,0.,1.));
#8258=DIRECTION('ref_axis',(1.,0.,0.));
#8259=DIRECTION('center_axis',(0.,-1.,0.));
#8260=DIRECTION('ref_axis',(0.,0.,-1.));
#8261=DIRECTION('center_axis',(0.,1.,0.));
#8262=DIRECTION('ref_axis',(1.,0.,0.));
#8263=DIRECTION('center_axis',(0.,-1.,0.));
#8264=DIRECTION('ref_axis',(1.,0.,0.));
#8265=DIRECTION('center_axis',(0.,-1.,0.));
#8266=DIRECTION('ref_axis',(0.,0.,-1.));
#8267=DIRECTION('center_axis',(0.,0.,1.));
#8268=DIRECTION('ref_axis',(1.,0.,0.));
#8269=DIRECTION('center_axis',(0.,-1.,0.));
#8270=DIRECTION('ref_axis',(0.,0.,-1.));
#8271=DIRECTION('center_axis',(0.,1.,0.));
#8272=DIRECTION('ref_axis',(1.,0.,0.));
#8273=DIRECTION('center_axis',(0.,-1.,0.));
#8274=DIRECTION('ref_axis',(1.,0.,0.));
#8275=DIRECTION('center_axis',(0.,-1.,0.));
#8276=DIRECTION('ref_axis',(0.,0.,-1.));
#8277=DIRECTION('center_axis',(6.12323399573676E-17,0.,1.));
#8278=DIRECTION('ref_axis',(1.,0.,0.));
#8279=DIRECTION('center_axis',(0.,-1.,0.));
#8280=DIRECTION('ref_axis',(0.,0.,-1.));
#8281=DIRECTION('center_axis',(0.,1.,0.));
#8282=DIRECTION('ref_axis',(1.,0.,0.));
#8283=DIRECTION('center_axis',(0.,-1.,0.));
#8284=DIRECTION('ref_axis',(1.,0.,0.));
#8285=DIRECTION('center_axis',(0.,-1.,0.));
#8286=DIRECTION('ref_axis',(0.,0.,-1.));
#8287=DIRECTION('center_axis',(0.,0.,1.));
#8288=DIRECTION('ref_axis',(1.,0.,0.));
#8289=DIRECTION('center_axis',(0.,-1.,0.));
#8290=DIRECTION('ref_axis',(0.,0.,-1.));
#8291=DIRECTION('center_axis',(0.,1.,0.));
#8292=DIRECTION('ref_axis',(1.,0.,0.));
#8293=DIRECTION('center_axis',(0.,1.,0.));
#8294=DIRECTION('ref_axis',(1.,0.,0.));
#8295=DIRECTION('',(0.,1.,0.));
#8296=DIRECTION('center_axis',(0.,-1.,0.));
#8297=DIRECTION('ref_axis',(1.,0.,0.));
#8298=DIRECTION('center_axis',(0.,-1.,0.));
#8299=DIRECTION('ref_axis',(1.,0.,0.));
#8300=DIRECTION('center_axis',(0.,1.,0.));
#8301=DIRECTION('ref_axis',(1.,0.,0.));
#8302=DIRECTION('center_axis',(0.,-1.,0.));
#8303=DIRECTION('ref_axis',(0.,0.,-1.));
#8304=DIRECTION('center_axis',(0.,0.,1.));
#8305=DIRECTION('ref_axis',(1.,0.,0.));
#8306=DIRECTION('center_axis',(0.,-1.,0.));
#8307=DIRECTION('ref_axis',(0.,0.,-1.));
#8308=DIRECTION('center_axis',(0.,-1.,0.));
#8309=DIRECTION('ref_axis',(-1.,0.,0.));
#8310=DIRECTION('center_axis',(0.,1.,0.));
#8311=DIRECTION('ref_axis',(1.,0.,0.));
#10270=CARTESIAN_POINT('',(0.,0.,0.));
#10271=CARTESIAN_POINT('Origin',(0.707106781186547,0.,0.707106781186548));
#10272=CARTESIAN_POINT('',(0.504455939115715,-0.04763,0.841298510752802));
#10273=CARTESIAN_POINT('',(0.841298510752802,-0.04763,0.504455939115715));
#10274=CARTESIAN_POINT('Ctrl Pts',(0.504455939115715,-0.04763,0.841298510752802));
#10275=CARTESIAN_POINT('Ctrl Pts',(0.508899795931835,-0.0740444353928835,
0.838633903678357));
#10276=CARTESIAN_POINT('Ctrl Pts',(0.517157748491652,-0.0999305678883309,
0.833661031856294));
#10277=CARTESIAN_POINT('Ctrl Pts',(0.537715343527944,-0.142345102874864,
0.820511285096538));
#10278=CARTESIAN_POINT('Ctrl Pts',(0.548874290046456,-0.159766064500479,
0.813159949759));
#10279=CARTESIAN_POINT('Ctrl Pts',(0.573915184558107,-0.190326085855194,
0.795684265985089));
#10280=CARTESIAN_POINT('Ctrl Pts',(0.587792702767295,-0.203463743702801,
0.78555112003688));
#10281=CARTESIAN_POINT('Ctrl Pts',(0.615966552324775,-0.224161999508995,
0.763642258217233));
#10282=CARTESIAN_POINT('Ctrl Pts',(0.631684198665438,-0.232861760990032,
0.750785745543687));
#10283=CARTESIAN_POINT('Ctrl Pts',(0.663382628119203,-0.244251601209411,
0.722929908501543));
#10284=CARTESIAN_POINT('Ctrl Pts',(0.679352081686668,-0.246942143572133,
0.707917883896095));
#10285=CARTESIAN_POINT('Ctrl Pts',(0.707917883896095,-0.246942143572133,
0.679352081686668));
#10286=CARTESIAN_POINT('Ctrl Pts',(0.722929908501543,-0.244251601209411,
0.663382628119203));
#10287=CARTESIAN_POINT('Ctrl Pts',(0.750785745543687,-0.232861760990032,
0.631684198665439));
#10288=CARTESIAN_POINT('Ctrl Pts',(0.763642258217232,-0.224161999508995,
0.615966552324775));
#10289=CARTESIAN_POINT('Ctrl Pts',(0.78555112003688,-0.203463743702801,
0.587792702767295));
#10290=CARTESIAN_POINT('Ctrl Pts',(0.795684265985088,-0.190326085855194,
0.573915184558108));
#10291=CARTESIAN_POINT('Ctrl Pts',(0.813159949759,-0.15976606450048,0.548874290046456));
#10292=CARTESIAN_POINT('Ctrl Pts',(0.820511285096538,-0.142345102874864,
0.537715343527944));
#10293=CARTESIAN_POINT('Ctrl Pts',(0.833661031856294,-0.099930567888331,
0.517157748491653));
#10294=CARTESIAN_POINT('Ctrl Pts',(0.838633903678357,-0.0740444353928835,
0.508899795931835));
#10295=CARTESIAN_POINT('Ctrl Pts',(0.841298510752801,-0.0476299999999999,
0.504455939115715));
#10296=CARTESIAN_POINT('',(0.528110872004958,-0.04763,0.871530771444223));
#10297=CARTESIAN_POINT('Origin',(0.707106781186547,-0.04763,0.707106781186548));
#10298=CARTESIAN_POINT('',(0.871530771444223,-0.04763,0.528110872004959));
#10299=CARTESIAN_POINT('Ctrl Pts',(0.871530771444223,-0.0476300000000001,
0.528110872004958));
#10300=CARTESIAN_POINT('Ctrl Pts',(0.87014664509073,-0.0609922781173483,
0.530395067942936));
#10301=CARTESIAN_POINT('Ctrl Pts',(0.868149331745851,-0.0742967091364493,
0.533674141594226));
#10302=CARTESIAN_POINT('Ctrl Pts',(0.85981294420286,-0.115492077056649,
0.54708917182331));
#10303=CARTESIAN_POINT('Ctrl Pts',(0.850993704737257,-0.141695629206859,
0.560922177770136));
#10304=CARTESIAN_POINT('Ctrl Pts',(0.830754510485543,-0.181890537957859,
0.590422647829571));
#10305=CARTESIAN_POINT('Ctrl Pts',(0.816896541396381,-0.201072148666545,
0.609616703125488));
#10306=CARTESIAN_POINT('Ctrl Pts',(0.792310597819928,-0.223955109275652,
0.641117951819998));
#10307=CARTESIAN_POINT('Ctrl Pts',(0.779109323683612,-0.232742381310829,
0.657208095763053));
#10308=CARTESIAN_POINT('Ctrl Pts',(0.750552691816206,-0.244234834628584,
0.68964083160521));
#10309=CARTESIAN_POINT('Ctrl Pts',(0.735185187071673,-0.246942143572133,
0.705971972091755));
#10310=CARTESIAN_POINT('Ctrl Pts',(0.705971972091754,-0.246942143572133,
0.735185187071673));
#10311=CARTESIAN_POINT('Ctrl Pts',(0.689640831605209,-0.244234834628584,
0.750552691816206));
#10312=CARTESIAN_POINT('Ctrl Pts',(0.657208095763052,-0.232742381310829,
0.779109323683612));
#10313=CARTESIAN_POINT('Ctrl Pts',(0.641117951819998,-0.223955109275652,
0.792310597819928));
#10314=CARTESIAN_POINT('Ctrl Pts',(0.609616703125487,-0.201072148666545,
0.816896541396382));
#10315=CARTESIAN_POINT('Ctrl Pts',(0.590422647829571,-0.181890537957858,
0.830754510485544));
#10316=CARTESIAN_POINT('Ctrl Pts',(0.560922177770135,-0.141695629206858,
0.850993704737257));
#10317=CARTESIAN_POINT('Ctrl Pts',(0.547089171823309,-0.115492077056649,
0.859812944202861));
#10318=CARTESIAN_POINT('Ctrl Pts',(0.533674141594226,-0.0742967091364491,
0.868149331745852));
#10319=CARTESIAN_POINT('Ctrl Pts',(0.530395067942936,-0.0609922781173483,
0.870146645090731));
#10320=CARTESIAN_POINT('Ctrl Pts',(0.528110872004958,-0.0476300000000001,
0.871530771444223));
#10321=CARTESIAN_POINT('Origin',(0.707106781186547,-0.04763,0.707106781186548));
#10322=CARTESIAN_POINT('Origin',(0.,-0.166705,0.));
#10323=CARTESIAN_POINT('',(0.242834539687906,-0.04763,0.989696097314));
#10324=CARTESIAN_POINT('Origin',(0.,-0.04763,0.));
#10325=CARTESIAN_POINT('',(-0.242834539687907,-0.04763,0.989696097314));
#10326=CARTESIAN_POINT('Ctrl Pts',(0.242834539687906,-0.04763,0.989696097314));
#10327=CARTESIAN_POINT('Ctrl Pts',(0.24024064412003,-0.0609922781173483,
0.990332542620729));
#10328=CARTESIAN_POINT('Ctrl Pts',(0.236509675094874,-0.0742967091364492,
0.991238884025248));
#10329=CARTESIAN_POINT('Ctrl Pts',(0.221129100087819,-0.115492077056649,
0.994830026707808));
#10330=CARTESIAN_POINT('Ctrl Pts',(0.205111543747588,-0.141695629206859,
0.998375294985966));
#10331=CARTESIAN_POINT('Ctrl Pts',(0.169940289819232,-0.181890537957859,
1.00492400591205));
#10332=CARTESIAN_POINT('Ctrl Pts',(0.1465689792446,-0.201072148666545,1.00869718865384));
#10333=CARTESIAN_POINT('Ctrl Pts',(0.106909345252087,-0.223955109275652,
1.01358704779679));
#10334=CARTESIAN_POINT('Ctrl Pts',(0.0861971848975941,-0.232742381310829,
1.0156297872271));
#10335=CARTESIAN_POINT('Ctrl Pts',(0.0430711894098822,-0.244234834628584,
1.01837060663223));
#10336=CARTESIAN_POINT('Ctrl Pts',(0.0206568624125605,-0.246942143572133,
1.019052));
#10337=CARTESIAN_POINT('Ctrl Pts',(-0.0206568624125608,-0.246942143572133,
1.019052));
#10338=CARTESIAN_POINT('Ctrl Pts',(-0.0430711894098825,-0.244234834628584,
1.01837060663223));
#10339=CARTESIAN_POINT('Ctrl Pts',(-0.0861971848975943,-0.232742381310829,
1.0156297872271));
#10340=CARTESIAN_POINT('Ctrl Pts',(-0.106909345252088,-0.223955109275652,
1.01358704779679));
#10341=CARTESIAN_POINT('Ctrl Pts',(-0.1465689792446,-0.201072148666545,
1.00869718865384));
#10342=CARTESIAN_POINT('Ctrl Pts',(-0.169940289819232,-0.181890537957859,
1.00492400591205));
#10343=CARTESIAN_POINT('Ctrl Pts',(-0.205111543747588,-0.141695629206859,
0.998375294985966));
#10344=CARTESIAN_POINT('Ctrl Pts',(-0.221129100087819,-0.115492077056649,
0.994830026707808));
#10345=CARTESIAN_POINT('Ctrl Pts',(-0.236509675094875,-0.0742967091364493,
0.991238884025248));
#10346=CARTESIAN_POINT('Ctrl Pts',(-0.24024064412003,-0.0609922781173483,
0.990332542620729));
#10347=CARTESIAN_POINT('Ctrl Pts',(-0.242834539687907,-0.04763,0.989696097314));
#10348=CARTESIAN_POINT('',(-0.528110872004959,-0.04763,0.871530771444223));
#10349=CARTESIAN_POINT('Origin',(0.,-0.04763,0.));
#10350=CARTESIAN_POINT('',(-0.871530771444223,-0.04763,0.528110872004958));
#10351=CARTESIAN_POINT('Ctrl Pts',(-0.528110872004958,-0.0476300000000001,
0.871530771444223));
#10352=CARTESIAN_POINT('Ctrl Pts',(-0.530395067942936,-0.0609922781173484,
0.87014664509073));
#10353=CARTESIAN_POINT('Ctrl Pts',(-0.533674141594226,-0.0742967091364493,
0.868149331745851));
#10354=CARTESIAN_POINT('Ctrl Pts',(-0.54708917182331,-0.115492077056649,
0.85981294420286));
#10355=CARTESIAN_POINT('Ctrl Pts',(-0.560922177770136,-0.141695629206859,
0.850993704737257));
#10356=CARTESIAN_POINT('Ctrl Pts',(-0.590422647829571,-0.181890537957859,
0.830754510485543));
#10357=CARTESIAN_POINT('Ctrl Pts',(-0.609616703125488,-0.201072148666545,
0.816896541396381));
#10358=CARTESIAN_POINT('Ctrl Pts',(-0.641117951819998,-0.223955109275652,
0.792310597819928));
#10359=CARTESIAN_POINT('Ctrl Pts',(-0.657208095763053,-0.232742381310829,
0.779109323683611));
#10360=CARTESIAN_POINT('Ctrl Pts',(-0.68964083160521,-0.244234834628584,
0.750552691816205));
#10361=CARTESIAN_POINT('Ctrl Pts',(-0.705971972091755,-0.246942143572133,
0.735185187071673));
#10362=CARTESIAN_POINT('Ctrl Pts',(-0.735185187071673,-0.246942143572133,
0.705971972091754));
#10363=CARTESIAN_POINT('Ctrl Pts',(-0.750552691816206,-0.244234834628584,
0.689640831605209));
#10364=CARTESIAN_POINT('Ctrl Pts',(-0.779109323683612,-0.232742381310829,
0.657208095763052));
#10365=CARTESIAN_POINT('Ctrl Pts',(-0.792310597819928,-0.223955109275652,
0.641117951819998));
#10366=CARTESIAN_POINT('Ctrl Pts',(-0.816896541396382,-0.201072148666545,
0.609616703125487));
#10367=CARTESIAN_POINT('Ctrl Pts',(-0.830754510485544,-0.181890537957858,
0.590422647829571));
#10368=CARTESIAN_POINT('Ctrl Pts',(-0.850993704737257,-0.141695629206858,
0.560922177770135));
#10369=CARTESIAN_POINT('Ctrl Pts',(-0.859812944202861,-0.115492077056649,
0.547089171823309));
#10370=CARTESIAN_POINT('Ctrl Pts',(-0.868149331745852,-0.0742967091364491,
0.533674141594226));
#10371=CARTESIAN_POINT('Ctrl Pts',(-0.870146645090731,-0.0609922781173483,
0.530395067942936));
#10372=CARTESIAN_POINT('Ctrl Pts',(-0.871530771444223,-0.04763,0.528110872004958));
#10373=CARTESIAN_POINT('',(-0.989696097314,-0.04763,0.242834539687906));
#10374=CARTESIAN_POINT('Origin',(0.,-0.04763,0.));
#10375=CARTESIAN_POINT('',(-1.019052,-0.246942143572133,1.248489836334E-16));
#10376=CARTESIAN_POINT('Ctrl Pts',(-0.989696097314,-0.04763,0.242834539687906));
#10377=CARTESIAN_POINT('Ctrl Pts',(-0.990332542620729,-0.0609922781173483,
0.24024064412003));
#10378=CARTESIAN_POINT('Ctrl Pts',(-0.991238884025248,-0.0742967091364492,
0.236509675094874));
#10379=CARTESIAN_POINT('Ctrl Pts',(-0.994830026707808,-0.115492077056649,
0.221129100087819));
#10380=CARTESIAN_POINT('Ctrl Pts',(-0.998375294985966,-0.141695629206859,
0.205111543747588));
#10381=CARTESIAN_POINT('Ctrl Pts',(-1.00492400591205,-0.181890537957859,
0.169940289819232));
#10382=CARTESIAN_POINT('Ctrl Pts',(-1.00869718865384,-0.201072148666545,
0.1465689792446));
#10383=CARTESIAN_POINT('Ctrl Pts',(-1.01358704779679,-0.223955109275652,
0.106909345252088));
#10384=CARTESIAN_POINT('Ctrl Pts',(-1.0156297872271,-0.232742381310829,
0.0861971848975944));
#10385=CARTESIAN_POINT('Ctrl Pts',(-1.01837060663223,-0.244234834628584,
0.0430711894098825));
#10386=CARTESIAN_POINT('Ctrl Pts',(-1.019052,-0.246942143572133,0.0206568624125608));
#10387=CARTESIAN_POINT('Ctrl Pts',(-1.019052,-0.246942143572133,1.2490009027033E-16));
#10388=CARTESIAN_POINT('',(-1.019052,-0.28578,1.24797876996471E-16));
#10389=CARTESIAN_POINT('',(-1.019052,-0.166705,1.24797876996471E-16));
#10390=CARTESIAN_POINT('Origin',(0.,-0.28578,0.));
#10391=CARTESIAN_POINT('',(-0.989696097314,-0.04763,-0.242834539687906));
#10392=CARTESIAN_POINT('Ctrl Pts',(-1.019052,-0.246942143572133,1.2490009027033E-16));
#10393=CARTESIAN_POINT('Ctrl Pts',(-1.019052,-0.246942143572133,-0.0206568624125605));
#10394=CARTESIAN_POINT('Ctrl Pts',(-1.01837060663223,-0.244234834628584,
-0.0430711894098822));
#10395=CARTESIAN_POINT('Ctrl Pts',(-1.0156297872271,-0.232742381310829,
-0.0861971848975941));
#10396=CARTESIAN_POINT('Ctrl Pts',(-1.01358704779679,-0.223955109275652,
-0.106909345252087));
#10397=CARTESIAN_POINT('Ctrl Pts',(-1.00869718865384,-0.201072148666546,
-0.1465689792446));
#10398=CARTESIAN_POINT('Ctrl Pts',(-1.00492400591205,-0.181890537957859,
-0.169940289819232));
#10399=CARTESIAN_POINT('Ctrl Pts',(-0.998375294985966,-0.141695629206859,
-0.205111543747588));
#10400=CARTESIAN_POINT('Ctrl Pts',(-0.994830026707808,-0.11549207705665,
-0.221129100087819));
#10401=CARTESIAN_POINT('Ctrl Pts',(-0.991238884025248,-0.0742967091364495,
-0.236509675094874));
#10402=CARTESIAN_POINT('Ctrl Pts',(-0.990332542620729,-0.0609922781173484,
-0.24024064412003));
#10403=CARTESIAN_POINT('Ctrl Pts',(-0.989696097314,-0.0476300000000001,
-0.242834539687907));
#10404=CARTESIAN_POINT('',(-0.871530771444223,-0.04763,-0.528110872004958));
#10405=CARTESIAN_POINT('Origin',(0.,-0.04763,0.));
#10406=CARTESIAN_POINT('',(-0.528110872004958,-0.04763,-0.871530771444223));
#10407=CARTESIAN_POINT('Ctrl Pts',(-0.871530771444223,-0.0476300000000001,
-0.528110872004958));
#10408=CARTESIAN_POINT('Ctrl Pts',(-0.87014664509073,-0.0609922781173484,
-0.530395067942936));
#10409=CARTESIAN_POINT('Ctrl Pts',(-0.868149331745851,-0.0742967091364494,
-0.533674141594226));
#10410=CARTESIAN_POINT('Ctrl Pts',(-0.85981294420286,-0.115492077056649,
-0.54708917182331));
#10411=CARTESIAN_POINT('Ctrl Pts',(-0.850993704737257,-0.141695629206859,
-0.560922177770136));
#10412=CARTESIAN_POINT('Ctrl Pts',(-0.830754510485543,-0.181890537957859,
-0.590422647829571));
#10413=CARTESIAN_POINT('Ctrl Pts',(-0.816896541396381,-0.201072148666546,
-0.609616703125488));
#10414=CARTESIAN_POINT('Ctrl Pts',(-0.792310597819928,-0.223955109275652,
-0.641117951819999));
#10415=CARTESIAN_POINT('Ctrl Pts',(-0.779109323683611,-0.232742381310829,
-0.657208095763053));
#10416=CARTESIAN_POINT('Ctrl Pts',(-0.750552691816205,-0.244234834628584,
-0.68964083160521));
#10417=CARTESIAN_POINT('Ctrl Pts',(-0.735185187071673,-0.246942143572133,
-0.705971972091755));
#10418=CARTESIAN_POINT('Ctrl Pts',(-0.705971972091754,-0.246942143572133,
-0.735185187071673));
#10419=CARTESIAN_POINT('Ctrl Pts',(-0.68964083160521,-0.244234834628584,
-0.750552691816206));
#10420=CARTESIAN_POINT('Ctrl Pts',(-0.657208095763052,-0.232742381310829,
-0.779109323683612));
#10421=CARTESIAN_POINT('Ctrl Pts',(-0.641117951819998,-0.223955109275652,
-0.792310597819928));
#10422=CARTESIAN_POINT('Ctrl Pts',(-0.609616703125488,-0.201072148666545,
-0.816896541396381));
#10423=CARTESIAN_POINT('Ctrl Pts',(-0.590422647829571,-0.181890537957859,
-0.830754510485543));
#10424=CARTESIAN_POINT('Ctrl Pts',(-0.560922177770136,-0.141695629206859,
-0.850993704737257));
#10425=CARTESIAN_POINT('Ctrl Pts',(-0.54708917182331,-0.115492077056649,
-0.85981294420286));
#10426=CARTESIAN_POINT('Ctrl Pts',(-0.533674141594226,-0.0742967091364494,
-0.868149331745852));
#10427=CARTESIAN_POINT('Ctrl Pts',(-0.530395067942936,-0.0609922781173484,
-0.870146645090731));
#10428=CARTESIAN_POINT('Ctrl Pts',(-0.528110872004958,-0.0476300000000001,
-0.871530771444223));
#10429=CARTESIAN_POINT('',(-0.242834539687906,-0.04763,-0.989696097314));
#10430=CARTESIAN_POINT('Origin',(0.,-0.04763,0.));
#10431=CARTESIAN_POINT('',(0.242834539687906,-0.04763,-0.989696097314));
#10432=CARTESIAN_POINT('Ctrl Pts',(-0.242834539687907,-0.04763,-0.989696097314));
#10433=CARTESIAN_POINT('Ctrl Pts',(-0.24024064412003,-0.0609922781173483,
-0.990332542620729));
#10434=CARTESIAN_POINT('Ctrl Pts',(-0.236509675094874,-0.0742967091364493,
-0.991238884025248));
#10435=CARTESIAN_POINT('Ctrl Pts',(-0.221129100087819,-0.115492077056649,
-0.994830026707808));
#10436=CARTESIAN_POINT('Ctrl Pts',(-0.205111543747588,-0.141695629206859,
-0.998375294985966));
#10437=CARTESIAN_POINT('Ctrl Pts',(-0.169940289819232,-0.181890537957859,
-1.00492400591205));
#10438=CARTESIAN_POINT('Ctrl Pts',(-0.1465689792446,-0.201072148666545,
-1.00869718865384));
#10439=CARTESIAN_POINT('Ctrl Pts',(-0.106909345252087,-0.223955109275652,
-1.01358704779679));
#10440=CARTESIAN_POINT('Ctrl Pts',(-0.0861971848975942,-0.232742381310829,
-1.0156297872271));
#10441=CARTESIAN_POINT('Ctrl Pts',(-0.0430711894098823,-0.244234834628584,
-1.01837060663223));
#10442=CARTESIAN_POINT('Ctrl Pts',(-0.0206568624125606,-0.246942143572133,
-1.019052));
#10443=CARTESIAN_POINT('Ctrl Pts',(0.0206568624125607,-0.246942143572133,
-1.019052));
#10444=CARTESIAN_POINT('Ctrl Pts',(0.0430711894098824,-0.244234834628584,
-1.01837060663223));
#10445=CARTESIAN_POINT('Ctrl Pts',(0.0861971848975943,-0.232742381310829,
-1.0156297872271));
#10446=CARTESIAN_POINT('Ctrl Pts',(0.106909345252088,-0.223955109275652,
-1.01358704779679));
#10447=CARTESIAN_POINT('Ctrl Pts',(0.1465689792446,-0.201072148666545,-1.00869718865384));
#10448=CARTESIAN_POINT('Ctrl Pts',(0.169940289819232,-0.181890537957859,
-1.00492400591205));
#10449=CARTESIAN_POINT('Ctrl Pts',(0.205111543747588,-0.141695629206859,
-0.998375294985966));
#10450=CARTESIAN_POINT('Ctrl Pts',(0.221129100087819,-0.115492077056649,
-0.994830026707808));
#10451=CARTESIAN_POINT('Ctrl Pts',(0.236509675094874,-0.0742967091364493,
-0.991238884025248));
#10452=CARTESIAN_POINT('Ctrl Pts',(0.24024064412003,-0.0609922781173484,
-0.990332542620729));
#10453=CARTESIAN_POINT('Ctrl Pts',(0.242834539687907,-0.04763,-0.989696097314));
#10454=CARTESIAN_POINT('',(0.528110872004958,-0.04763,-0.871530771444223));
#10455=CARTESIAN_POINT('Origin',(0.,-0.04763,0.));
#10456=CARTESIAN_POINT('',(0.871530771444223,-0.04763,-0.528110872004958));
#10457=CARTESIAN_POINT('Ctrl Pts',(0.528110872004958,-0.0476300000000001,
-0.871530771444223));
#10458=CARTESIAN_POINT('Ctrl Pts',(0.530395067942936,-0.0609922781173484,
-0.870146645090731));
#10459=CARTESIAN_POINT('Ctrl Pts',(0.533674141594226,-0.0742967091364493,
-0.868149331745851));
#10460=CARTESIAN_POINT('Ctrl Pts',(0.54708917182331,-0.115492077056649,
-0.85981294420286));
#10461=CARTESIAN_POINT('Ctrl Pts',(0.560922177770136,-0.141695629206859,
-0.850993704737257));
#10462=CARTESIAN_POINT('Ctrl Pts',(0.590422647829571,-0.181890537957859,
-0.830754510485543));
#10463=CARTESIAN_POINT('Ctrl Pts',(0.609616703125488,-0.201072148666545,
-0.816896541396381));
#10464=CARTESIAN_POINT('Ctrl Pts',(0.641117951819998,-0.223955109275652,
-0.792310597819928));
#10465=CARTESIAN_POINT('Ctrl Pts',(0.657208095763053,-0.232742381310829,
-0.779109323683612));
#10466=CARTESIAN_POINT('Ctrl Pts',(0.68964083160521,-0.244234834628584,
-0.750552691816206));
#10467=CARTESIAN_POINT('Ctrl Pts',(0.705971972091755,-0.246942143572133,
-0.735185187071673));
#10468=CARTESIAN_POINT('Ctrl Pts',(0.735185187071673,-0.246942143572133,
-0.705971972091754));
#10469=CARTESIAN_POINT('Ctrl Pts',(0.750552691816206,-0.244234834628584,
-0.68964083160521));
#10470=CARTESIAN_POINT('Ctrl Pts',(0.779109323683612,-0.232742381310829,
-0.657208095763053));
#10471=CARTESIAN_POINT('Ctrl Pts',(0.792310597819928,-0.223955109275652,
-0.641117951819998));
#10472=CARTESIAN_POINT('Ctrl Pts',(0.816896541396381,-0.201072148666545,
-0.609616703125488));
#10473=CARTESIAN_POINT('Ctrl Pts',(0.830754510485543,-0.181890537957859,
-0.590422647829571));
#10474=CARTESIAN_POINT('Ctrl Pts',(0.850993704737257,-0.141695629206859,
-0.560922177770136));
#10475=CARTESIAN_POINT('Ctrl Pts',(0.85981294420286,-0.115492077056649,
-0.54708917182331));
#10476=CARTESIAN_POINT('Ctrl Pts',(0.868149331745851,-0.0742967091364493,
-0.533674141594226));
#10477=CARTESIAN_POINT('Ctrl Pts',(0.870146645090731,-0.0609922781173484,
-0.530395067942936));
#10478=CARTESIAN_POINT('Ctrl Pts',(0.871530771444223,-0.0476300000000001,
-0.528110872004958));
#10479=CARTESIAN_POINT('',(0.989696097314,-0.04763,-0.242834539687906));
#10480=CARTESIAN_POINT('Origin',(0.,-0.04763,0.));
#10481=CARTESIAN_POINT('',(0.989696097314,-0.04763,0.242834539687906));
#10482=CARTESIAN_POINT('Ctrl Pts',(0.989696097314,-0.04763,-0.242834539687907));
#10483=CARTESIAN_POINT('Ctrl Pts',(0.990332542620729,-0.0609922781173483,
-0.24024064412003));
#10484=CARTESIAN_POINT('Ctrl Pts',(0.991238884025248,-0.0742967091364493,
-0.236509675094874));
#10485=CARTESIAN_POINT('Ctrl Pts',(0.994830026707808,-0.115492077056649,
-0.221129100087819));
#10486=CARTESIAN_POINT('Ctrl Pts',(0.998375294985966,-0.141695629206859,
-0.205111543747588));
#10487=CARTESIAN_POINT('Ctrl Pts',(1.00492400591205,-0.181890537957859,
-0.169940289819232));
#10488=CARTESIAN_POINT('Ctrl Pts',(1.00869718865384,-0.201072148666545,
-0.1465689792446));
#10489=CARTESIAN_POINT('Ctrl Pts',(1.01358704779679,-0.223955109275652,
-0.106909345252087));
#10490=CARTESIAN_POINT('Ctrl Pts',(1.0156297872271,-0.232742381310829,-0.0861971848975942));
#10491=CARTESIAN_POINT('Ctrl Pts',(1.01837060663223,-0.244234834628584,
-0.0430711894098823));
#10492=CARTESIAN_POINT('Ctrl Pts',(1.019052,-0.246942143572133,-0.0206568624125607));
#10493=CARTESIAN_POINT('Ctrl Pts',(1.019052,-0.246942143572133,0.0206568624125607));
#10494=CARTESIAN_POINT('Ctrl Pts',(1.01837060663223,-0.244234834628584,
0.0430711894098823));
#10495=CARTESIAN_POINT('Ctrl Pts',(1.0156297872271,-0.232742381310829,0.0861971848975942));
#10496=CARTESIAN_POINT('Ctrl Pts',(1.01358704779679,-0.223955109275652,
0.106909345252087));
#10497=CARTESIAN_POINT('Ctrl Pts',(1.00869718865384,-0.201072148666545,
0.1465689792446));
#10498=CARTESIAN_POINT('Ctrl Pts',(1.00492400591205,-0.181890537957859,
0.169940289819232));
#10499=CARTESIAN_POINT('Ctrl Pts',(0.998375294985966,-0.141695629206859,
0.205111543747588));
#10500=CARTESIAN_POINT('Ctrl Pts',(0.994830026707808,-0.115492077056649,
0.221129100087819));
#10501=CARTESIAN_POINT('Ctrl Pts',(0.991238884025248,-0.0742967091364492,
0.236509675094874));
#10502=CARTESIAN_POINT('Ctrl Pts',(0.990332542620729,-0.0609922781173483,
0.24024064412003));
#10503=CARTESIAN_POINT('Ctrl Pts',(0.989696097314,-0.04763,0.242834539687907));
#10504=CARTESIAN_POINT('Origin',(0.,-0.04763,0.));
#10505=CARTESIAN_POINT('Origin',(0.,-0.04763,0.));
#10506=CARTESIAN_POINT('',(0.238183666596899,-0.04763,0.951592097314));
#10507=CARTESIAN_POINT('Origin',(0.,-0.04763,0.));
#10508=CARTESIAN_POINT('Origin',(-1.94289029309402E-16,-0.04763,1.));
#10509=CARTESIAN_POINT('Origin',(-1.94289029309402E-16,0.,1.));
#10510=CARTESIAN_POINT('',(-0.2381836665969,-0.04763,0.951592097314));
#10511=CARTESIAN_POINT('Ctrl Pts',(-0.238183666596899,-0.0476299999999999,
0.951592097314));
#10512=CARTESIAN_POINT('Ctrl Pts',(-0.233157223576062,-0.0740444353928835,
0.952850216871763));
#10513=CARTESIAN_POINT('Ctrl Pts',(-0.223801617934946,-0.0999305678883309,
0.955173119738174));
#10514=CARTESIAN_POINT('Ctrl Pts',(-0.199966927975188,-0.142345102874864,
0.960411259488514));
#10515=CARTESIAN_POINT('Ctrl Pts',(-0.1868781821531,-0.159766064500479,
0.963103647174702));
#10516=CARTESIAN_POINT('Ctrl Pts',(-0.15681442133453,-0.190326085855194,
0.968453058988463));
#10517=CARTESIAN_POINT('Ctrl Pts',(-0.139836317888043,-0.203463743702801,
0.971100730005489));
#10518=CARTESIAN_POINT('Ctrl Pts',(-0.104422493053067,-0.224161999508995,
0.975530745318961));
#10519=CARTESIAN_POINT('Ctrl Pts',(-0.0842175114474176,-0.232861760990032,
0.977553872336861));
#10520=CARTESIAN_POINT('Ctrl Pts',(-0.0421062857595701,-0.244251601209411,
0.980270995488453));
#10521=CARTESIAN_POINT('Ctrl Pts',(-0.0201990724523197,-0.246942143572133,
0.980948));
#10522=CARTESIAN_POINT('Ctrl Pts',(0.020199072452319,-0.246942143572133,
0.980948));
#10523=CARTESIAN_POINT('Ctrl Pts',(0.0421062857595694,-0.244251601209411,
0.980270995488454));
#10524=CARTESIAN_POINT('Ctrl Pts',(0.0842175114474169,-0.232861760990032,
0.977553872336861));
#10525=CARTESIAN_POINT('Ctrl Pts',(0.104422493053067,-0.224161999508995,
0.975530745318961));
#10526=CARTESIAN_POINT('Ctrl Pts',(0.139836317888042,-0.203463743702801,
0.971100730005489));
#10527=CARTESIAN_POINT('Ctrl Pts',(0.15681442133453,-0.190326085855194,
0.968453058988463));
#10528=CARTESIAN_POINT('Ctrl Pts',(0.1868781821531,-0.15976606450048,0.963103647174702));
#10529=CARTESIAN_POINT('Ctrl Pts',(0.199966927975188,-0.142345102874864,
0.960411259488514));
#10530=CARTESIAN_POINT('Ctrl Pts',(0.223801617934945,-0.0999305678883309,
0.955173119738174));
#10531=CARTESIAN_POINT('Ctrl Pts',(0.233157223576061,-0.0740444353928835,
0.952850216871763));
#10532=CARTESIAN_POINT('Ctrl Pts',(0.238183666596899,-0.0476299999999999,
0.951592097314));
#10533=CARTESIAN_POINT('Origin',(-1.94289029309402E-16,-0.04763,1.));
#10534=CARTESIAN_POINT('Origin',(0.,-0.04763,0.));
#10535=CARTESIAN_POINT('',(-0.504455939115715,-0.04763,0.841298510752802));
#10536=CARTESIAN_POINT('Origin',(0.,-0.04763,0.));
#10537=CARTESIAN_POINT('Origin',(-0.707106781186548,-0.04763,0.707106781186547));
#10538=CARTESIAN_POINT('Origin',(-0.707106781186548,0.,0.707106781186547));
#10539=CARTESIAN_POINT('',(-0.841298510752802,-0.04763,0.504455939115715));
#10540=CARTESIAN_POINT('Ctrl Pts',(-0.841298510752802,-0.04763,0.504455939115715));
#10541=CARTESIAN_POINT('Ctrl Pts',(-0.838633903678357,-0.0740444353928835,
0.508899795931835));
#10542=CARTESIAN_POINT('Ctrl Pts',(-0.833661031856294,-0.0999305678883309,
0.517157748491652));
#10543=CARTESIAN_POINT('Ctrl Pts',(-0.820511285096538,-0.142345102874864,
0.537715343527944));
#10544=CARTESIAN_POINT('Ctrl Pts',(-0.813159949759,-0.159766064500479,0.548874290046456));
#10545=CARTESIAN_POINT('Ctrl Pts',(-0.795684265985089,-0.190326085855194,
0.573915184558107));
#10546=CARTESIAN_POINT('Ctrl Pts',(-0.78555112003688,-0.203463743702801,
0.587792702767295));
#10547=CARTESIAN_POINT('Ctrl Pts',(-0.763642258217233,-0.224161999508995,
0.615966552324775));
#10548=CARTESIAN_POINT('Ctrl Pts',(-0.750785745543687,-0.232861760990032,
0.631684198665438));
#10549=CARTESIAN_POINT('Ctrl Pts',(-0.722929908501543,-0.244251601209411,
0.663382628119203));
#10550=CARTESIAN_POINT('Ctrl Pts',(-0.707917883896095,-0.246942143572133,
0.679352081686668));
#10551=CARTESIAN_POINT('Ctrl Pts',(-0.679352081686668,-0.246942143572133,
0.707917883896095));
#10552=CARTESIAN_POINT('Ctrl Pts',(-0.663382628119203,-0.244251601209411,
0.722929908501544));
#10553=CARTESIAN_POINT('Ctrl Pts',(-0.631684198665438,-0.232861760990031,
0.750785745543687));
#10554=CARTESIAN_POINT('Ctrl Pts',(-0.615966552324775,-0.224161999508995,
0.763642258217233));
#10555=CARTESIAN_POINT('Ctrl Pts',(-0.587792702767295,-0.203463743702801,
0.78555112003688));
#10556=CARTESIAN_POINT('Ctrl Pts',(-0.573915184558107,-0.190326085855194,
0.795684265985088));
#10557=CARTESIAN_POINT('Ctrl Pts',(-0.548874290046456,-0.159766064500479,
0.813159949759));
#10558=CARTESIAN_POINT('Ctrl Pts',(-0.537715343527944,-0.142345102874864,
0.820511285096538));
#10559=CARTESIAN_POINT('Ctrl Pts',(-0.517157748491652,-0.0999305678883309,
0.833661031856294));
#10560=CARTESIAN_POINT('Ctrl Pts',(-0.508899795931835,-0.0740444353928835,
0.838633903678357));
#10561=CARTESIAN_POINT('Ctrl Pts',(-0.504455939115716,-0.04763,0.841298510752801));
#10562=CARTESIAN_POINT('Origin',(-0.707106781186548,-0.04763,0.707106781186547));
#10563=CARTESIAN_POINT('Origin',(0.,-0.04763,0.));
#10564=CARTESIAN_POINT('',(-0.951592097314,-0.04763,0.238183666596899));
#10565=CARTESIAN_POINT('Origin',(0.,-0.04763,0.));
#10566=CARTESIAN_POINT('Origin',(-1.,-0.04763,-1.11022302462516E-16));
#10567=CARTESIAN_POINT('Origin',(-1.,0.,-1.11022302462516E-16));
#10568=CARTESIAN_POINT('',(-0.951592097314,-0.04763,-0.2381836665969));
#10569=CARTESIAN_POINT('',(-0.980948,-0.246942143572133,1.08514323328844E-18));
#10570=CARTESIAN_POINT('Ctrl Pts',(-0.951592097314,-0.04763,-0.238183666596899));
#10571=CARTESIAN_POINT('Ctrl Pts',(-0.952850216871763,-0.0740444353928835,
-0.233157223576062));
#10572=CARTESIAN_POINT('Ctrl Pts',(-0.955173119738174,-0.0999305678883309,
-0.223801617934946));
#10573=CARTESIAN_POINT('Ctrl Pts',(-0.960411259488514,-0.142345102874864,
-0.199966927975188));
#10574=CARTESIAN_POINT('Ctrl Pts',(-0.963103647174702,-0.159766064500479,
-0.1868781821531));
#10575=CARTESIAN_POINT('Ctrl Pts',(-0.968453058988463,-0.190326085855194,
-0.15681442133453));
#10576=CARTESIAN_POINT('Ctrl Pts',(-0.971100730005489,-0.203463743702801,
-0.139836317888043));
#10577=CARTESIAN_POINT('Ctrl Pts',(-0.975530745318961,-0.224161999508995,
-0.104422493053067));
#10578=CARTESIAN_POINT('Ctrl Pts',(-0.977553872336861,-0.232861760990032,
-0.0842175114474175));
#10579=CARTESIAN_POINT('Ctrl Pts',(-0.980270995488453,-0.244251601209411,
-0.0421062857595699));
#10580=CARTESIAN_POINT('Ctrl Pts',(-0.980948,-0.246942143572133,-0.0201990724523195));
#10581=CARTESIAN_POINT('Ctrl Pts',(-0.980948,-0.246942143572133,-1.17961196366423E-16));
#10582=CARTESIAN_POINT('Origin',(-1.,-0.04763,-1.11022302462516E-16));
#10583=CARTESIAN_POINT('Ctrl Pts',(-0.980948,-0.246942143572133,-1.17961196366423E-16));
#10584=CARTESIAN_POINT('Ctrl Pts',(-0.980948,-0.246942143572133,0.0201990724523192));
#10585=CARTESIAN_POINT('Ctrl Pts',(-0.980270995488453,-0.244251601209411,
0.0421062857595695));
#10586=CARTESIAN_POINT('Ctrl Pts',(-0.977553872336861,-0.232861760990032,
0.0842175114474169));
#10587=CARTESIAN_POINT('Ctrl Pts',(-0.975530745318961,-0.224161999508995,
0.104422493053066));
#10588=CARTESIAN_POINT('Ctrl Pts',(-0.971100730005489,-0.203463743702801,
0.139836317888042));
#10589=CARTESIAN_POINT('Ctrl Pts',(-0.968453058988463,-0.190326085855194,
0.15681442133453));
#10590=CARTESIAN_POINT('Ctrl Pts',(-0.963103647174702,-0.15976606450048,
0.1868781821531));
#10591=CARTESIAN_POINT('Ctrl Pts',(-0.960411259488514,-0.142345102874864,
0.199966927975188));
#10592=CARTESIAN_POINT('Ctrl Pts',(-0.955173119738174,-0.099930567888331,
0.223801617934945));
#10593=CARTESIAN_POINT('Ctrl Pts',(-0.952850216871763,-0.0740444353928835,
0.233157223576061));
#10594=CARTESIAN_POINT('Ctrl Pts',(-0.951592097314,-0.04763,0.238183666596899));
#10595=CARTESIAN_POINT('Origin',(0.,-0.04763,0.));
#10596=CARTESIAN_POINT('',(-0.841298510752802,-0.04763,-0.504455939115715));
#10597=CARTESIAN_POINT('Origin',(0.,-0.04763,0.));
#10598=CARTESIAN_POINT('Origin',(-0.707106781186547,-0.04763,-0.707106781186548));
#10599=CARTESIAN_POINT('Origin',(-0.707106781186547,0.,-0.707106781186548));
#10600=CARTESIAN_POINT('',(-0.504455939115715,-0.04763,-0.841298510752802));
#10601=CARTESIAN_POINT('Ctrl Pts',(-0.504455939115715,-0.04763,-0.841298510752802));
#10602=CARTESIAN_POINT('Ctrl Pts',(-0.508899795931835,-0.0740444353928835,
-0.838633903678357));
#10603=CARTESIAN_POINT('Ctrl Pts',(-0.517157748491652,-0.0999305678883309,
-0.833661031856294));
#10604=CARTESIAN_POINT('Ctrl Pts',(-0.537715343527944,-0.142345102874864,
-0.820511285096538));
#10605=CARTESIAN_POINT('Ctrl Pts',(-0.548874290046456,-0.159766064500479,
-0.813159949759));
#10606=CARTESIAN_POINT('Ctrl Pts',(-0.573915184558107,-0.190326085855194,
-0.795684265985089));
#10607=CARTESIAN_POINT('Ctrl Pts',(-0.587792702767295,-0.203463743702801,
-0.78555112003688));
#10608=CARTESIAN_POINT('Ctrl Pts',(-0.615966552324775,-0.224161999508995,
-0.763642258217233));
#10609=CARTESIAN_POINT('Ctrl Pts',(-0.631684198665438,-0.232861760990032,
-0.750785745543687));
#10610=CARTESIAN_POINT('Ctrl Pts',(-0.663382628119203,-0.244251601209411,
-0.722929908501543));
#10611=CARTESIAN_POINT('Ctrl Pts',(-0.679352081686668,-0.246942143572133,
-0.707917883896095));
#10612=CARTESIAN_POINT('Ctrl Pts',(-0.707917883896095,-0.246942143572133,
-0.679352081686668));
#10613=CARTESIAN_POINT('Ctrl Pts',(-0.722929908501543,-0.244251601209411,
-0.663382628119203));
#10614=CARTESIAN_POINT('Ctrl Pts',(-0.750785745543687,-0.232861760990032,
-0.631684198665439));
#10615=CARTESIAN_POINT('Ctrl Pts',(-0.763642258217232,-0.224161999508995,
-0.615966552324775));
#10616=CARTESIAN_POINT('Ctrl Pts',(-0.78555112003688,-0.203463743702801,
-0.587792702767295));
#10617=CARTESIAN_POINT('Ctrl Pts',(-0.795684265985088,-0.190326085855194,
-0.573915184558107));
#10618=CARTESIAN_POINT('Ctrl Pts',(-0.813159949759,-0.15976606450048,-0.548874290046456));
#10619=CARTESIAN_POINT('Ctrl Pts',(-0.820511285096538,-0.142345102874864,
-0.537715343527944));
#10620=CARTESIAN_POINT('Ctrl Pts',(-0.833661031856294,-0.0999305678883311,
-0.517157748491652));
#10621=CARTESIAN_POINT('Ctrl Pts',(-0.838633903678357,-0.0740444353928836,
-0.508899795931835));
#10622=CARTESIAN_POINT('Ctrl Pts',(-0.841298510752801,-0.04763,-0.504455939115715));
#10623=CARTESIAN_POINT('Origin',(-0.707106781186547,-0.04763,-0.707106781186548));
#10624=CARTESIAN_POINT('Origin',(0.,-0.04763,0.));
#10625=CARTESIAN_POINT('',(-0.238183666596899,-0.04763,-0.951592097314));
#10626=CARTESIAN_POINT('Origin',(0.,-0.04763,0.));
#10627=CARTESIAN_POINT('Origin',(5.55111512312578E-17,-0.04763,-1.));
#10628=CARTESIAN_POINT('Origin',(5.55111512312578E-17,0.,-1.));
#10629=CARTESIAN_POINT('',(0.238183666596899,-0.04763,-0.951592097314));
#10630=CARTESIAN_POINT('Ctrl Pts',(0.238183666596899,-0.04763,-0.951592097314));
#10631=CARTESIAN_POINT('Ctrl Pts',(0.233157223576062,-0.0740444353928835,
-0.952850216871763));
#10632=CARTESIAN_POINT('Ctrl Pts',(0.223801617934946,-0.099930567888331,
-0.955173119738174));
#10633=CARTESIAN_POINT('Ctrl Pts',(0.199966927975188,-0.142345102874864,
-0.960411259488514));
#10634=CARTESIAN_POINT('Ctrl Pts',(0.1868781821531,-0.15976606450048,-0.963103647174702));
#10635=CARTESIAN_POINT('Ctrl Pts',(0.15681442133453,-0.190326085855194,
-0.968453058988463));
#10636=CARTESIAN_POINT('Ctrl Pts',(0.139836317888042,-0.203463743702801,
-0.971100730005489));
#10637=CARTESIAN_POINT('Ctrl Pts',(0.104422493053067,-0.224161999508995,
-0.975530745318961));
#10638=CARTESIAN_POINT('Ctrl Pts',(0.0842175114474173,-0.232861760990032,
-0.977553872336861));
#10639=CARTESIAN_POINT('Ctrl Pts',(0.0421062857595698,-0.244251601209411,
-0.980270995488453));
#10640=CARTESIAN_POINT('Ctrl Pts',(0.0201990724523194,-0.246942143572133,
-0.980948));
#10641=CARTESIAN_POINT('Ctrl Pts',(-0.0201990724523193,-0.246942143572133,
-0.980948));
#10642=CARTESIAN_POINT('Ctrl Pts',(-0.0421062857595697,-0.244251601209411,
-0.980270995488453));
#10643=CARTESIAN_POINT('Ctrl Pts',(-0.0842175114474171,-0.232861760990032,
-0.977553872336861));
#10644=CARTESIAN_POINT('Ctrl Pts',(-0.104422493053067,-0.224161999508995,
-0.975530745318961));
#10645=CARTESIAN_POINT('Ctrl Pts',(-0.139836317888042,-0.203463743702801,
-0.971100730005489));
#10646=CARTESIAN_POINT('Ctrl Pts',(-0.15681442133453,-0.190326085855194,
-0.968453058988463));
#10647=CARTESIAN_POINT('Ctrl Pts',(-0.1868781821531,-0.15976606450048,-0.963103647174702));
#10648=CARTESIAN_POINT('Ctrl Pts',(-0.199966927975188,-0.142345102874864,
-0.960411259488514));
#10649=CARTESIAN_POINT('Ctrl Pts',(-0.223801617934945,-0.099930567888331,
-0.955173119738174));
#10650=CARTESIAN_POINT('Ctrl Pts',(-0.233157223576062,-0.0740444353928835,
-0.952850216871763));
#10651=CARTESIAN_POINT('Ctrl Pts',(-0.238183666596899,-0.0476299999999999,
-0.951592097314));
#10652=CARTESIAN_POINT('Origin',(5.55111512312578E-17,-0.04763,-1.));
#10653=CARTESIAN_POINT('Origin',(0.,-0.04763,0.));
#10654=CARTESIAN_POINT('',(0.504455939115715,-0.04763,-0.841298510752802));
#10655=CARTESIAN_POINT('Origin',(0.,-0.04763,0.));
#10656=CARTESIAN_POINT('Origin',(0.707106781186548,-0.04763,-0.707106781186547));
#10657=CARTESIAN_POINT('Origin',(0.707106781186548,0.,-0.707106781186547));
#10658=CARTESIAN_POINT('',(0.841298510752802,-0.04763,-0.504455939115715));
#10659=CARTESIAN_POINT('Ctrl Pts',(0.841298510752802,-0.04763,-0.504455939115715));
#10660=CARTESIAN_POINT('Ctrl Pts',(0.838633903678357,-0.0740444353928835,
-0.508899795931835));
#10661=CARTESIAN_POINT('Ctrl Pts',(0.833661031856294,-0.0999305678883309,
-0.517157748491652));
#10662=CARTESIAN_POINT('Ctrl Pts',(0.820511285096538,-0.142345102874864,
-0.537715343527944));
#10663=CARTESIAN_POINT('Ctrl Pts',(0.813159949759,-0.159766064500479,-0.548874290046456));
#10664=CARTESIAN_POINT('Ctrl Pts',(0.795684265985088,-0.190326085855194,
-0.573915184558107));
#10665=CARTESIAN_POINT('Ctrl Pts',(0.78555112003688,-0.203463743702801,
-0.587792702767295));
#10666=CARTESIAN_POINT('Ctrl Pts',(0.763642258217233,-0.224161999508995,
-0.615966552324775));
#10667=CARTESIAN_POINT('Ctrl Pts',(0.750785745543687,-0.232861760990032,
-0.631684198665438));
#10668=CARTESIAN_POINT('Ctrl Pts',(0.722929908501543,-0.244251601209411,
-0.663382628119203));
#10669=CARTESIAN_POINT('Ctrl Pts',(0.707917883896095,-0.246942143572133,
-0.679352081686668));
#10670=CARTESIAN_POINT('Ctrl Pts',(0.679352081686668,-0.246942143572133,
-0.707917883896095));
#10671=CARTESIAN_POINT('Ctrl Pts',(0.663382628119203,-0.244251601209411,
-0.722929908501543));
#10672=CARTESIAN_POINT('Ctrl Pts',(0.631684198665438,-0.232861760990032,
-0.750785745543687));
#10673=CARTESIAN_POINT('Ctrl Pts',(0.615966552324775,-0.224161999508995,
-0.763642258217232));
#10674=CARTESIAN_POINT('Ctrl Pts',(0.587792702767295,-0.203463743702801,
-0.78555112003688));
#10675=CARTESIAN_POINT('Ctrl Pts',(0.573915184558107,-0.190326085855194,
-0.795684265985088));
#10676=CARTESIAN_POINT('Ctrl Pts',(0.548874290046456,-0.159766064500479,
-0.813159949759));
#10677=CARTESIAN_POINT('Ctrl Pts',(0.537715343527944,-0.142345102874864,
-0.820511285096538));
#10678=CARTESIAN_POINT('Ctrl Pts',(0.517157748491652,-0.099930567888331,
-0.833661031856294));
#10679=CARTESIAN_POINT('Ctrl Pts',(0.508899795931835,-0.0740444353928835,
-0.838633903678357));
#10680=CARTESIAN_POINT('Ctrl Pts',(0.504455939115715,-0.04763,-0.841298510752801));
#10681=CARTESIAN_POINT('Origin',(0.707106781186548,-0.04763,-0.707106781186547));
#10682=CARTESIAN_POINT('Origin',(0.,-0.166705,0.));
#10683=CARTESIAN_POINT('',(-0.980948,-0.28578,1.20131482833E-16));
#10684=CARTESIAN_POINT('Origin',(0.,-0.28578,0.));
#10685=CARTESIAN_POINT('',(-0.980948,-0.166705,1.20131482833E-16));
#10686=CARTESIAN_POINT('',(0.951592097314,-0.04763,0.238183666596899));
#10687=CARTESIAN_POINT('Origin',(0.,-0.04763,0.));
#10688=CARTESIAN_POINT('',(0.951592097314,-0.04763,-0.238183666596899));
#10689=CARTESIAN_POINT('Ctrl Pts',(0.951592097314,-0.04763,0.238183666596899));
#10690=CARTESIAN_POINT('Ctrl Pts',(0.952850216871763,-0.0740444353928835,
0.233157223576062));
#10691=CARTESIAN_POINT('Ctrl Pts',(0.955173119738174,-0.099930567888331,
0.223801617934945));
#10692=CARTESIAN_POINT('Ctrl Pts',(0.960411259488514,-0.142345102874864,
0.199966927975188));
#10693=CARTESIAN_POINT('Ctrl Pts',(0.963103647174702,-0.15976606450048,
0.1868781821531));
#10694=CARTESIAN_POINT('Ctrl Pts',(0.968453058988463,-0.190326085855194,
0.15681442133453));
#10695=CARTESIAN_POINT('Ctrl Pts',(0.971100730005489,-0.203463743702801,
0.139836317888042));
#10696=CARTESIAN_POINT('Ctrl Pts',(0.975530745318961,-0.224161999508995,
0.104422493053067));
#10697=CARTESIAN_POINT('Ctrl Pts',(0.977553872336861,-0.232861760990032,
0.0842175114474172));
#10698=CARTESIAN_POINT('Ctrl Pts',(0.980270995488453,-0.244251601209411,
0.0421062857595697));
#10699=CARTESIAN_POINT('Ctrl Pts',(0.980948,-0.246942143572133,0.0201990724523194));
#10700=CARTESIAN_POINT('Ctrl Pts',(0.980948,-0.246942143572133,-0.0201990724523194));
#10701=CARTESIAN_POINT('Ctrl Pts',(0.980270995488453,-0.244251601209411,
-0.0421062857595697));
#10702=CARTESIAN_POINT('Ctrl Pts',(0.977553872336861,-0.232861760990032,
-0.0842175114474172));
#10703=CARTESIAN_POINT('Ctrl Pts',(0.975530745318961,-0.224161999508995,
-0.104422493053067));
#10704=CARTESIAN_POINT('Ctrl Pts',(0.971100730005489,-0.203463743702801,
-0.139836317888042));
#10705=CARTESIAN_POINT('Ctrl Pts',(0.968453058988463,-0.190326085855194,
-0.15681442133453));
#10706=CARTESIAN_POINT('Ctrl Pts',(0.963103647174702,-0.15976606450048,
-0.1868781821531));
#10707=CARTESIAN_POINT('Ctrl Pts',(0.960411259488514,-0.142345102874864,
-0.199966927975188));
#10708=CARTESIAN_POINT('Ctrl Pts',(0.955173119738174,-0.099930567888331,
-0.223801617934945));
#10709=CARTESIAN_POINT('Ctrl Pts',(0.952850216871763,-0.0740444353928835,
-0.233157223576062));
#10710=CARTESIAN_POINT('Ctrl Pts',(0.951592097314,-0.0476299999999999,-0.238183666596899));
#10711=CARTESIAN_POINT('Origin',(0.,-0.04763,0.));
#10712=CARTESIAN_POINT('Origin',(0.,-0.04763,0.));
#10713=CARTESIAN_POINT('Origin',(1.,-0.04763,0.));
#10714=CARTESIAN_POINT('Origin',(1.,0.,0.));
#10715=CARTESIAN_POINT('Origin',(1.,-0.04763,0.));
#10716=CARTESIAN_POINT('Origin',(0.,-0.28578,0.));
#10717=CARTESIAN_POINT('Origin',(0.,-0.04763,0.));
#11838=UNCERTAINTY_MEASURE_WITH_UNIT(LENGTH_MEASURE(0.001),#11917,
'DISTANCE_ACCURACY_VALUE',
'Maximum model space distance between geometric entities at asserted c
onnectivities');
#11869=UNCERTAINTY_MEASURE_WITH_UNIT(LENGTH_MEASURE(0.001),#11917,
'DISTANCE_ACCURACY_VALUE',
'Maximum model space distance between geometric entities at asserted c
onnectivities');
#11885=(
GEOMETRIC_REPRESENTATION_CONTEXT(3)
GLOBAL_UNCERTAINTY_ASSIGNED_CONTEXT((#11838))
GLOBAL_UNIT_ASSIGNED_CONTEXT((#11917,#11919,#11920))
REPRESENTATION_CONTEXT('','3D')
);
#11916=(
GEOMETRIC_REPRESENTATION_CONTEXT(3)
GLOBAL_UNCERTAINTY_ASSIGNED_CONTEXT((#11869))
GLOBAL_UNIT_ASSIGNED_CONTEXT((#11917,#11919,#11920))
REPRESENTATION_CONTEXT('','3D')
);
#11917=(
LENGTH_UNIT()
NAMED_UNIT(*)
SI_UNIT(.CENTI.,.METRE.)
);
#11919=(
NAMED_UNIT(*)
PLANE_ANGLE_UNIT()
SI_UNIT($,.RADIAN.)
);
#11920=(
NAMED_UNIT(*)
SI_UNIT($,.STERADIAN.)
SOLID_ANGLE_UNIT()
);
#11936=SHAPE_DEFINITION_REPRESENTATION(#11982,#12094);
#11982=PRODUCT_DEFINITION_SHAPE('',$,#12141);
#12094=SHAPE_REPRESENTATION('',(#6887),#11885);
#12125=PRODUCT_DEFINITION_CONTEXT('part definition',#12265,'design');
#12141=PRODUCT_DEFINITION('Cage','Cage',#12187,#12125);
#12187=PRODUCT_DEFINITION_FORMATION('',$,#12282);
#12265=APPLICATION_CONTEXT(
'Core Data for Automotive Mechanical Design Process');
#12266=PRODUCT_CONTEXT('part definition',#12265,'mechanical');
#12282=PRODUCT('Cage','Cage','Cage',(#12266));
#12369=COLOUR_RGB('Grey',0.48,0.52,0.57);
#12370=FILL_AREA_STYLE_COLOUR('',#12369);
#12371=FILL_AREA_STYLE('',(#12370));
#12372=SURFACE_STYLE_FILL_AREA(#12371);
#12373=SURFACE_SIDE_STYLE('',(#12372));
#12374=SURFACE_STYLE_USAGE(.BOTH.,#12373);
#12375=PRESENTATION_STYLE_ASSIGNMENT((#12374));
ENDSEC;
END-ISO-10303-21;
